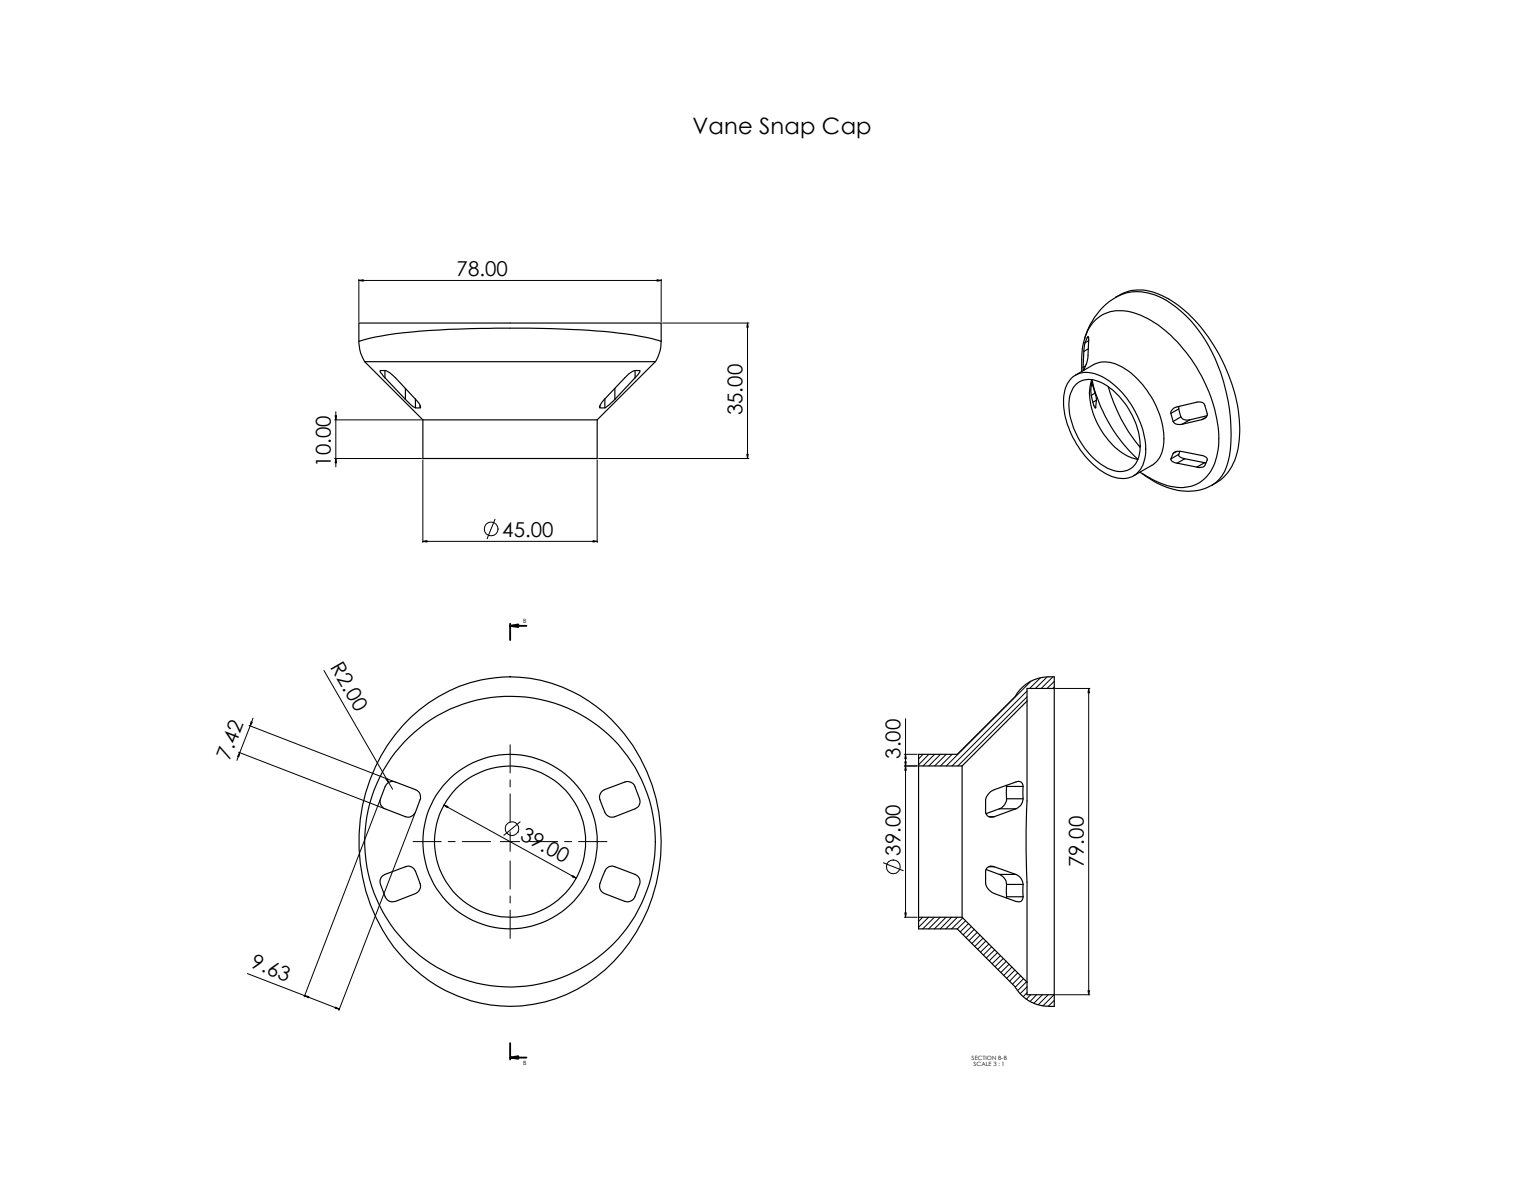
ISO-10303-21;
HEADER;
FILE_DESCRIPTION (('STEP AP214'),
    '1' );
FILE_NAME ('Vane Snap Cap.step',
    '2026-10-18T20:16:25',
    ( '' ),
    ( '' ),
    'SwSTEP 2.0',
    'SolidWorks 2025',
    '' );
FILE_SCHEMA (( 'AUTOMOTIVE_DESIGN' ));
ENDSEC;

DATA;
#5=CARTESIAN_POINT ( 'NONE',  ( -18.15804816958924306, -34.11099862341368549, 27.50000000000000000 ) ) ;
#9=CARTESIAN_POINT ( 'NONE',  ( -8.101746394734353984, -38.49011865887880646, 34.49999999999998579 ) ) ;
#19=CARTESIAN_POINT ( 'NONE',  ( 24.39344986792568903, -29.07448411189255211, 27.50000000000001066 ) ) ;
#42=EDGE_CURVE ( 'NONE', #19602, #22873, #7666, .T. ) ;
#47=CARTESIAN_POINT ( 'NONE',  ( 36.14613918203227172, 16.01870328439765601, 34.83083827288849221 ) ) ;
#98=CARTESIAN_POINT ( 'NONE',  ( -37.93368909164158254, 9.961195697873989729, 34.97277436636965575 ) ) ;
#131=CARTESIAN_POINT ( 'NONE',  ( 23.21352257770656635, -10.78826658734920052, 45.15942333309103418 ) ) ;
#132=ORIENTED_EDGE ( 'NONE', *, *, #23307, .F. ) ;
#138=AXIS2_PLACEMENT_3D ( 'NONE', #523, #22041, #27196 ) ;
#155=CARTESIAN_POINT ( 'NONE',  ( -7.108788511070779137, -38.72574257930638453, 34.49999999999999289 ) ) ;
#165=VERTEX_POINT ( 'NONE', #8736 ) ;
#166=CARTESIAN_POINT ( 'NONE',  ( 22.55938241427807256, 30.80590877286595841, 27.50000000000000355 ) ) ;
#170=DIRECTION ( 'NONE',  ( -0.000000000000000000, -0.000000000000000000, 1.000000000000000000 ) ) ;
#171=CARTESIAN_POINT ( 'NONE',  ( -30.03865005752669148, 15.52610542268208604, 41.18623755349101856 ) ) ;
#177=ORIENTED_EDGE ( 'NONE', *, *, #24246, .F. ) ;
#188=CARTESIAN_POINT ( 'NONE',  ( 27.51850911855329329, 30.14776422306135117, 30.03356538881464743 ) ) ;
#215=CARTESIAN_POINT ( 'NONE',  ( 24.35970437652574105, 13.37404834226503958, 47.21042702067963859 ) ) ;
#217=CARTESIAN_POINT ( 'NONE',  ( 19.49999999999992539, 1.626584906615178899E-14, 62.49999999999999289 ) ) ;
#224=B_SPLINE_CURVE_WITH_KNOTS ( 'NONE', 3,
 ( #24253, #10067, #7738, #5394 ),
 .UNSPECIFIED., .F., .F.,
 ( 4, 4 ),
 ( 2.143643656977390230E-07, 0.003421830178490235883 ),
 .UNSPECIFIED. ) ;
#247=CARTESIAN_POINT ( 'NONE',  ( -36.79585557548701757, 7.262324983800692912, 37.49999999996946087 ) ) ;
#254=VERTEX_POINT ( 'NONE', #21492 ) ;
#289=CARTESIAN_POINT ( 'NONE',  ( -32.19782014694307293, -14.25394737442115733, 39.78814634291943264 ) ) ;
#295=CARTESIAN_POINT ( 'NONE',  ( 25.24511578250132260, -28.23443549260979779, 34.49999999999999289 ) ) ;
#303=DIRECTION ( 'NONE',  ( 0.9329908884337535513, 0.3598999890241665334, 0.000000000000000000 ) ) ;
#309=CARTESIAN_POINT ( 'NONE',  ( -8.593763153356288598, -38.36129777999322954, 34.49999999999998579 ) ) ;
#338=CARTESIAN_POINT ( 'NONE',  ( 37.49999999999997158, 1.387778780781445676E-14, 37.50000000000000000 ) ) ;
#344=CARTESIAN_POINT ( 'NONE',  ( 30.96653510607171711, 25.84892707844779736, 34.59766498189470241 ) ) ;
#361=CARTESIAN_POINT ( 'NONE',  ( -23.13350093726293366, 11.03024450687078861, 49.37167574286524996 ) ) ;
#365=ORIENTED_EDGE ( 'NONE', *, *, #16572, .F. ) ;
#403=CARTESIAN_POINT ( 'NONE',  ( 29.61203839202722676, 15.40012917324034092, 41.62281023987512185 ) ) ;
#404=CARTESIAN_POINT ( 'NONE',  ( -34.20659985760524080, -15.57190080006868271, 37.50000000004849454 ) ) ;
#438=VERTEX_POINT ( 'NONE', #18642 ) ;
#441=CARTESIAN_POINT ( 'NONE',  ( -26.81381729043377504, 6.366069288663346093, 47.44085139292785414 ) ) ;
#451=CARTESIAN_POINT ( 'NONE',  ( 5.060094141397912360, 42.14075867279367316, 28.87075318537527835 ) ) ;
#457=CARTESIAN_POINT ( 'NONE',  ( -37.32236259411956780, 12.59516552021271885, 31.74041422182562755 ) ) ;
#490=CARTESIAN_POINT ( 'NONE',  ( 34.70577939417254498, 10.49309206032065944, 34.49999999999999289 ) ) ;
#492=CARTESIAN_POINT ( 'NONE',  ( 30.03792366816882975, 15.52577997660843145, 41.18702913624200335 ) ) ;
#501=CARTESIAN_POINT ( 'NONE',  ( -24.35970437652574105, -13.37404834226503070, 47.21042702067970254 ) ) ;
#505=CARTESIAN_POINT ( 'NONE',  ( 34.07302093592694803, 20.85404585400097233, 34.70738523996037372 ) ) ;
#506=FACE_OUTER_BOUND ( 'NONE', #20914, .T. ) ;
#519=CARTESIAN_POINT ( 'NONE',  ( -10.95918588188520282, 37.64010906258869227, 34.49999999999998579 ) ) ;
#523=CARTESIAN_POINT ( 'NONE',  ( 24.44496207165490276, 7.595930209050162141, -16.55003854064094426 ) ) ;
#526=VERTEX_POINT ( 'NONE', #217 ) ;
#548=CARTESIAN_POINT ( 'NONE',  ( -32.31395967786516366, -23.80510233529698993, 30.69444703814347264 ) ) ;
#551=EDGE_CURVE ( 'NONE', #10953, #254, #7134, .T. ) ;
#587=EDGE_CURVE ( 'NONE', #12561, #19716, #26583, .T. ) ;
#591=CARTESIAN_POINT ( 'NONE',  ( 35.02974205252522211, 18.72736911740413746, 31.20071108243496738 ) ) ;
#598=CARTESIAN_POINT ( 'NONE',  ( -19.51604255644980412, 36.82188910226315670, 29.35984054749004102 ) ) ;
#603=B_SPLINE_CURVE_WITH_KNOTS ( 'NONE', 3,
 ( #9449, #13968, #2105, #21117 ),
 .UNSPECIFIED., .F., .F.,
 ( 4, 4 ),
 ( 0.002976194933398900420, 0.003711256114093792156 ),
 .UNSPECIFIED. ) ;
#627=FACE_OUTER_BOUND ( 'NONE', #19855, .T. ) ;
#631=VECTOR ( 'NONE', #12349, 1000.000000000000000 ) ;
#639=CARTESIAN_POINT ( 'NONE',  ( -34.70577939417217550, -10.49309206032214270, 34.49999999999999289 ) ) ;
#641=CARTESIAN_POINT ( 'NONE',  ( 33.50775388423620882, 10.82565592554877121, 39.78708271175815270 ) ) ;
#643=CARTESIAN_POINT ( 'NONE',  ( 26.12638453225886792, 6.310846377660611850, 48.12226976367801257 ) ) ;
#646=ORIENTED_EDGE ( 'NONE', *, *, #6616, .F. ) ;
#654=CARTESIAN_POINT ( 'NONE',  ( -23.21352257770656990, 10.78826658734919519, 45.15942333309111234 ) ) ;
#665=ORIENTED_EDGE ( 'NONE', *, *, #13448, .F. ) ;
#672=DIRECTION ( 'NONE',  ( 0.000000000000000000, 0.000000000000000000, 1.000000000000000000 ) ) ;
#673=AXIS2_PLACEMENT_3D ( 'NONE', #16914, #18794, #7091 ) ;
#691=ADVANCED_FACE ( 'NONE', ( #10356 ), #20168, .F. ) ;
#704=CARTESIAN_POINT ( 'NONE',  ( -23.18616900178304974, -34.18096212676299217, 29.62072393548881877 ) ) ;
#711=B_SPLINE_SURFACE_WITH_KNOTS ( 'NONE', 3, 1, ( 
 ( #29500, #24966 ),
 ( #10153, #22316 ),
 ( #12970, #26861 ),
 ( #19658, #19825 ),
 ( #29347, #17492 ),
 ( #14986, #8137 ),
 ( #24498, #17804 ),
 ( #8288, #19982 ),
 ( #27013, #3144 ),
 ( #22160, #10468 ),
 ( #22462, #1109 ),
 ( #3602, #784 ),
 ( #13124, #18259 ),
 ( #11231, #13728 ),
 ( #25438, #4063 ),
 ( #25586, #13590 ),
 ( #6246, #3761 ),
 ( #8739, #20888 ),
 ( #1268, #1716 ),
 ( #28075, #25729 ),
 ( #13882, #4358 ),
 ( #11397, #10776 ),
 ( #4204, #20290 ),
 ( #29817, #23067 ),
 ( #8905, #23219 ),
 ( #1579, #27470 ),
 ( #11086, #8459 ),
 ( #17959, #22774 ),
 ( #15601, #25119 ),
 ( #18429, #1873 ),
 ( #8599, #18107 ),
 ( #30107, #3924 ),
 ( #27622, #15755 ),
 ( #25276, #20582 ) ),
 .UNSPECIFIED., .F., .F., .F.,
 ( 4, 2, 2, 2, 2, 2, 2, 2, 2, 2, 2, 2, 2, 2, 2, 2, 4 ),
 ( 2, 2 ),
 ( 0.000000000000000000, 0.06250000000000008327, 0.1250000000000001388, 0.1875000000000001943, 0.2500000000000002220, 0.3125000000000002220, 0.3750000000000002776, 0.4375000000000002776, 0.5000000000000003331, 0.5625000000000003331, 0.6250000000000002220, 0.6875000000000002220, 0.7500000000000002220, 0.8125000000000002220, 0.8750000000000001110, 0.9375000000000001110, 1.000000000000000000 ),
 ( 0.000000000000000000, 1.000000000000000000 ),
 .UNSPECIFIED. ) ;
#718=ORIENTED_EDGE ( 'NONE', *, *, #23326, .F. ) ;
#727=CARTESIAN_POINT ( 'NONE',  ( -1.248051566150084613, -39.49999999999997158, 27.49999999999999289 ) ) ;
#738=CARTESIAN_POINT ( 'NONE',  ( 0.000000000000000000, 39.50000000000000000, 27.50000000000000355 ) ) ;
#744=CARTESIAN_POINT ( 'NONE',  ( -27.80440265630350538, 29.80991922482741785, 30.06891749665959779 ) ) ;
#745=CARTESIAN_POINT ( 'NONE',  ( 77.99999999999998579, 42.50000000000000711, 27.50000000000000711 ) ) ;
#749=CARTESIAN_POINT ( 'NONE',  ( 27.81206575847386375, -25.09777039261014053, 34.50000000000000711 ) ) ;
#772=EDGE_LOOP ( 'NONE', ( #4852, #18862, #30452, #1067 ) ) ;
#776=CARTESIAN_POINT ( 'NONE',  ( 24.35970437652574105, 13.37404834226503958, -16.55003854064094426 ) ) ;
#784=CARTESIAN_POINT ( 'NONE',  ( -31.18890335284658732, 19.89223002944919116, 27.50000000000001066 ) ) ;
#786=CARTESIAN_POINT ( 'NONE',  ( 30.86161751192252822, 15.46691422980913266, 40.47962024281689963 ) ) ;
#790=CARTESIAN_POINT ( 'NONE',  ( 26.58938213246210580, 6.321715805855840031, 47.66948656093867243 ) ) ;
#807=EDGE_CURVE ( 'NONE', #6797, #17083, #20091, .T. ) ;
#824=CARTESIAN_POINT ( 'NONE',  ( -15.61095767114878541, 35.65786817450091206, 34.50000000000000000 ) ) ;
#838=EDGE_CURVE ( 'NONE', #18044, #17963, #995, .T. ) ;
#842=LINE ( 'NONE', #3035, #21019 ) ;
#846=VECTOR ( 'NONE', #2060, 1000.000000000000000 ) ;
#849=CARTESIAN_POINT ( 'NONE',  ( -23.21352257770656990, -10.78826658734919519, 45.15942333309109813 ) ) ;
#862=CARTESIAN_POINT ( 'NONE',  ( -34.80856967755993736, -19.21184172954434999, 31.15481810886020497 ) ) ;
#906=CARTESIAN_POINT ( 'NONE',  ( 27.03074382657074537, 6.449748410230989215, -16.55003854064094426 ) ) ;
#918=CARTESIAN_POINT ( 'NONE',  ( -38.56714466680799802, -6.442804806652034699, 32.09716166004417914 ) ) ;
#942=EDGE_CURVE ( 'NONE', #28122, #2953, #17667, .T. ) ;
#948=CARTESIAN_POINT ( 'NONE',  ( 31.89304216768362821, -14.79375299452194170, 35.60059606544044186 ) ) ;
#954=CARTESIAN_POINT ( 'NONE',  ( 24.44496207165490276, 7.595930209050162141, 49.40206402021032517 ) ) ;
#956=CARTESIAN_POINT ( 'NONE',  ( 16.53285166946374929, 35.10262665635723778, 34.50000000000000000 ) ) ;
#960=CARTESIAN_POINT ( 'NONE',  ( 30.74147208807243103, 15.49548351932574874, 40.57409041152969564 ) ) ;
#961=ORIENTED_EDGE ( 'NONE', *, *, #13499, .F. ) ;
#965=CARTESIAN_POINT ( 'NONE',  ( 33.50775388423620882, 10.82565592554877121, 35.54444202463886882 ) ) ;
#975=CARTESIAN_POINT ( 'NONE',  ( 77.99999999999998579, -42.50000000000001421, 27.50000000000000711 ) ) ;
#976=CARTESIAN_POINT ( 'NONE',  ( 7.864568376310370645, 41.74085412114251881, 28.90542812248210325 ) ) ;
#979=CARTESIAN_POINT ( 'NONE',  ( 26.12638453225886792, 6.310846377660614515, 43.87962907655873579 ) ) ;
#989=CARTESIAN_POINT ( 'NONE',  ( -33.70208146031188789, 13.89198562565741923, 34.49999999999999289 ) ) ;
#995=B_SPLINE_CURVE_WITH_KNOTS ( 'NONE', 3,
 ( #11129, #20628, #30146, #15962, #30750, #9393, #21536, #24028, #23883, #14206, #14058, #171, #16252, #4861 ),
 .UNSPECIFIED., .F., .F.,
 ( 4, 2, 2, 2, 2, 2, 4 ),
 ( 2.111077618484504239E-07, 0.0004668847438969890226, 0.0009335583800321295943, 0.001400232016167270166, 0.001866905652302410738, 0.002800252924572703590, 0.003733600196842996443 ),
 .UNSPECIFIED. ) ;
#1006=EDGE_CURVE ( 'NONE', #20257, #22873, #4629, .T. ) ;
#1025=EDGE_CURVE ( 'NONE', #30101, #30448, #12431, .T. ) ;
#1026=CARTESIAN_POINT ( 'NONE',  ( -28.50858587296695745, -29.13344744256045615, 30.13847653714394070 ) ) ;
#1031=DIRECTION ( 'NONE',  ( -0.9329908884337535513, 0.3598999890241665334, 0.000000000000000000 ) ) ;
#1039=CIRCLE ( 'NONE', #2525, 19.49999999999996447 ) ;
#1048=VERTEX_POINT ( 'NONE', #5486 ) ;
#1067=ORIENTED_EDGE ( 'NONE', *, *, #3732, .F. ) ;
#1071=CARTESIAN_POINT ( 'NONE',  ( 25.56256718580103637, -32.12586005794658206, 29.82918954436054193 ) ) ;
#1103=CARTESIAN_POINT ( 'NONE',  ( -33.01877980957529957, 12.12572312222180493, 39.84356070656661331 ) ) ;
#1109=CARTESIAN_POINT ( 'NONE',  ( -28.55068628633582861, 24.19494186940698199, 27.50000000000001066 ) ) ;
#1117=LINE ( 'NONE', #9899, #29855 ) ;
#1125=CARTESIAN_POINT ( 'NONE',  ( 13.29126524260693998, 35.08562276291469573, 37.49999999993516298 ) ) ;
#1127=CARTESIAN_POINT ( 'NONE',  ( 24.44496207165490276, 7.595930209050162141, 45.15942333309104129 ) ) ;
#1129=DIRECTION ( 'NONE',  ( 1.000000000000000000, 0.000000000000000000, 0.000000000000000000 ) ) ;
#1144=FACE_OUTER_BOUND ( 'NONE', #21557, .T. ) ;
#1169=CARTESIAN_POINT ( 'NONE',  ( 24.35970437652574105, 13.37404834226503958, 42.96778633356035471 ) ) ;
#1179=CARTESIAN_POINT ( 'NONE',  ( -15.55309275218070830, -34.20504001467671884, 37.49999999988268229 ) ) ;
#1201=CARTESIAN_POINT ( 'NONE',  ( 33.26787633654601706, -9.290711110048576415, 40.45924760685198862 ) ) ;
#1203=VERTEX_POINT ( 'NONE', #29467 ) ;
#1210=EDGE_CURVE ( 'NONE', #27501, #29565, #30630, .T. ) ;
#1218=CARTESIAN_POINT ( 'NONE',  ( -4.163336342344337027E-14, 1.387778780781445676E-14, 37.50000000000000000 ) ) ;
#1229=CARTESIAN_POINT ( 'NONE',  ( -24.35970437652574105, 13.37404834226503247, 42.96778633356043287 ) ) ;
#1233=DIRECTION ( 'NONE',  ( 1.000000000000000000, 0.000000000000000000, 0.000000000000000000 ) ) ;
#1268=CARTESIAN_POINT ( 'NONE',  ( -35.76481447503398670, -5.202797454133643917, 34.80090346875804386 ) ) ;
#1269=CARTESIAN_POINT ( 'NONE',  ( 30.33183837007556249, 13.53414739637283226, -16.55003854064094426 ) ) ;
#1280=B_SPLINE_CURVE_WITH_KNOTS ( 'NONE', 3,
 ( #2307, #12145, #11993, #11834, #4507, #21164, #4800, #28524, #26026, #24132, #7155, #9957, #441, #2624 ),
 .UNSPECIFIED., .F., .F.,
 ( 4, 2, 2, 2, 2, 2, 4 ),
 ( 2.108610145898612731E-07, 0.0004867403503157787643, 0.0009732698396169676622, 0.001459799328918156506, 0.001946328818219345350, 0.002919387796821717399, 0.003892446775424089015 ),
 .UNSPECIFIED. ) ;
#1285=CARTESIAN_POINT ( 'NONE',  ( 19.84998497291395125, 36.59036391654254317, 29.38252776222237372 ) ) ;
#1287=CARTESIAN_POINT ( 'NONE',  ( -33.51229671200703564, -9.872960191568498800, 35.82118098709739940 ) ) ;
#1288=CARTESIAN_POINT ( 'NONE',  ( -33.48612972047447300, 10.91418318924902131, 39.78046893947538365 ) ) ;
#1296=CARTESIAN_POINT ( 'NONE',  ( 9.743151247090292344, -38.04912300944125292, 27.50000000000000000 ) ) ;
#1307=CARTESIAN_POINT ( 'NONE',  ( -24.44496207165490276, -7.595930209050158588, 49.40206402021039622 ) ) ;
#1309=B_SPLINE_CURVE_WITH_KNOTS ( 'NONE', 3,
 ( #28103, #25755, #20466, #11254 ),
 .UNSPECIFIED., .F., .F.,
 ( 4, 4 ),
 ( 3.022186913359086288E-07, 0.007932103869840195776 ),
 .UNSPECIFIED. ) ;
#1321=CARTESIAN_POINT ( 'NONE',  ( 27.86235613436985759, 14.72519157938689460, 39.24389099736750808 ) ) ;
#1326=CARTESIAN_POINT ( 'NONE',  ( -11.70595374688322821, -40.54787758647957219, 34.56692815348143455 ) ) ;
#1334=CARTESIAN_POINT ( 'NONE',  ( 31.89304216768362821, -14.79375299452194348, 39.84323675255973995 ) ) ;
#1336=ORIENTED_EDGE ( 'NONE', *, *, #9963, .T. ) ;
#1343=B_SPLINE_CURVE_WITH_KNOTS ( 'NONE', 3,
 ( #28708, #11874, #19499, #9676, #12175, #21673, #26843, #5148, #14659, #4840, #24161, #2813, #12336, #26205, #17153, #7650, #26672, #19039, #19641, #2509, #29011, #23697, #14510, #28553, #4998, #309, #9, #155, #7799, #14355, #12023, #7185, #23865, #21836 ),
 .UNSPECIFIED., .F., .F.,
 ( 4, 2, 2, 2, 2, 2, 2, 2, 2, 2, 2, 2, 2, 2, 2, 2, 4 ),
 ( 0.1877422973930296390, 0.1907727015327729259, 0.1938031056725162127, 0.1998639139520027586, 0.2028943180917460454, 0.2044095201616177027, 0.2059247222314893322, 0.2119855305109759058, 0.2150159346507191649, 0.2165311367205908222, 0.2180463387904624517, 0.2241071470699490531, 0.2271375512096923677, 0.2286527532795639972, 0.2301679553494356545, 0.2331983594891789413, 0.2362287636289222559 ),
 .UNSPECIFIED. ) ;
#1371=CARTESIAN_POINT ( 'NONE',  ( -5.974369479646943759, 42.02548368003539991, 34.60052964640640738 ) ) ;
#1384=CARTESIAN_POINT ( 'NONE',  ( 12.58101777923778997, -40.23389158998374171, 29.03989791324179848 ) ) ;
#1398=CARTESIAN_POINT ( 'NONE',  ( 35.99999999999999289, -2.601438916704202242, 34.80090346875810070 ) ) ;
#1412=CARTESIAN_POINT ( 'NONE',  ( 24.44496207165490276, -7.595930209050162141, -16.55003854064094426 ) ) ;
#1414=CARTESIAN_POINT ( 'NONE',  ( -33.43088607478084384, -9.613432587296607323, 40.21452297281935984 ) ) ;
#1439=ORIENTED_EDGE ( 'NONE', *, *, #14389, .F. ) ;
#1448=CYLINDRICAL_SURFACE ( 'NONE', #28363, 19.49999999999996447 ) ;
#1450=ORIENTED_EDGE ( 'NONE', *, *, #13936, .F. ) ;
#1452=CARTESIAN_POINT ( 'NONE',  ( -33.42925964089141644, -11.06161099612212695, 35.54550565580013455 ) ) ;
#1455=CARTESIAN_POINT ( 'NONE',  ( -33.42925964089140933, 11.06161099612212695, 39.78814634291943264 ) ) ;
#1474=PLANE ( 'NONE',  #26220 ) ;
#1483=CARTESIAN_POINT ( 'NONE',  ( 35.71656808851346199, -17.11898487263705704, 31.35097916509175420 ) ) ;
#1497=CARTESIAN_POINT ( 'NONE',  ( -31.10273980501929003, -15.38400267427140022, 40.30072466179765911 ) ) ;
#1511=CARTESIAN_POINT ( 'NONE',  ( 33.51208342369033488, -9.877893692955346694, 40.06259746622173168 ) ) ;
#1518=ORIENTED_EDGE ( 'NONE', *, *, #17633, .T. ) ;
#1526=CARTESIAN_POINT ( 'NONE',  ( -29.61203839202723032, -15.40012917324033381, 37.38016955275590192 ) ) ;
#1535=EDGE_LOOP ( 'NONE', ( #14556, #8831 ) ) ;
#1545=CARTESIAN_POINT ( 'NONE',  ( 17.94248964168179583, 34.33858135081683827, 34.80090346875809360 ) ) ;
#1547=ORIENTED_EDGE ( 'NONE', *, *, #7279, .F. ) ;
#1553=ORIENTED_EDGE ( 'NONE', *, *, #27298, .F. ) ;
#1558=CARTESIAN_POINT ( 'NONE',  ( 23.13152334643393715, 11.98019263786950184, 48.95036236640387983 ) ) ;
#1563=B_SPLINE_CURVE_WITH_KNOTS ( 'NONE', 3,
 ( #8926, #25745, #9067, #30722, #30123, #1889 ),
 .UNSPECIFIED., .F., .F.,
 ( 4, 2, 4 ),
 ( 0.01057608626842624147, 0.01589305904737019909, 0.02121003182631415324 ),
 .UNSPECIFIED. ) ;
#1575=CARTESIAN_POINT ( 'NONE',  ( 33.48319591361583036, 9.771272583783428445, 40.12028472023447279 ) ) ;
#1579=CARTESIAN_POINT ( 'NONE',  ( -23.69412710310941605, -29.84645176427128987, 34.80090346875804386 ) ) ;
#1597=EDGE_CURVE ( 'NONE', #6797, #18116, #28187, .T. ) ;
#1604=CARTESIAN_POINT ( 'NONE',  ( -33.03011559203990544, 8.976883822286589876, 40.77182279851235336 ) ) ;
#1607=ORIENTED_EDGE ( 'NONE', *, *, #15669, .T. ) ;
#1631=ORIENTED_EDGE ( 'NONE', *, *, #838, .F. ) ;
#1634=CARTESIAN_POINT ( 'NONE',  ( 35.57581530336350539, -17.46952725568587894, 34.79368316662617389 ) ) ;
#1636=VECTOR ( 'NONE', #26633, 1000.000000000000000 ) ;
#1669=CIRCLE ( 'NONE', #19099, 37.50000000000001421 ) ;
#1680=CARTESIAN_POINT ( 'NONE',  ( 31.34809375791739683, -25.29209928965034848, 30.54052050932160256 ) ) ;
#1681=DIRECTION ( 'NONE',  ( -0.000000000000000000, -0.000000000000000000, -1.000000000000000000 ) ) ;
#1698=CARTESIAN_POINT ( 'NONE',  ( -30.33183837007556249, -13.53414739637282516, -16.55003854064094426 ) ) ;
#1702=LINE ( 'NONE', #20570, #17967 ) ;
#1704=CARTESIAN_POINT ( 'NONE',  ( -23.07950435457407679, 11.50806656539752737, -16.55003854064094426 ) ) ;
#1708=ORIENTED_EDGE ( 'NONE', *, *, #23072, .F. ) ;
#1716=CARTESIAN_POINT ( 'NONE',  ( -35.76481447503398670, -5.202797454133643917, 27.50000000000000355 ) ) ;
#1733=ADVANCED_FACE ( 'NONE', ( #5565 ), #29631, .F. ) ;
#1734=CARTESIAN_POINT ( 'NONE',  ( 26.11179934312167816, -14.04991663536889135, 41.10667063058289727 ) ) ;
#1764=CARTESIAN_POINT ( 'NONE',  ( 32.19782014694307293, 14.25394737442116444, -16.55003854064094426 ) ) ;
#1775=CARTESIAN_POINT ( 'NONE',  ( 36.88240865182195449, -7.258209409195951700, 37.49999999993649880 ) ) ;
#1778=ORIENTED_EDGE ( 'NONE', *, *, #6616, .T. ) ;
#1784=VERTEX_POINT ( 'NONE', #4948 ) ;
#1786=CARTESIAN_POINT ( 'NONE',  ( -6.388525611213331068, -41.95271539343359990, 34.59875978651353989 ) ) ;
#1795=CARTESIAN_POINT ( 'NONE',  ( 23.07601128794333434, 11.40611796340042261, 45.01673140500131609 ) ) ;
#1802=CARTESIAN_POINT ( 'NONE',  ( 24.35970437652574816, -13.37404834226503958, 47.21042702067961727 ) ) ;
#1810=ORIENTED_EDGE ( 'NONE', *, *, #27747, .F. ) ;
#1823=ORIENTED_EDGE ( 'NONE', *, *, #26337, .F. ) ;
#1828=CARTESIAN_POINT ( 'NONE',  ( 29.61203839202725518, -15.40012917324033381, 41.62281023987508632 ) ) ;
#1839=CIRCLE ( 'NONE', #27764, 37.50000000000001421 ) ;
#1848=CARTESIAN_POINT ( 'NONE',  ( 17.94248964168179583, -34.33858135081684537, 34.80090346875808649 ) ) ;
#1873=CARTESIAN_POINT ( 'NONE',  ( -11.52197458429825261, -37.50933785548060229, 27.49999999999999645 ) ) ;
#1888=CARTESIAN_POINT ( 'NONE',  ( 0.000000000000000000, 42.50000000000000000, 37.50000000000000000 ) ) ;
#1889=CARTESIAN_POINT ( 'NONE',  ( 34.70577939417254498, 10.49309206032065944, 34.49999999999999289 ) ) ;
#1890=CARTESIAN_POINT ( 'NONE',  ( 24.35970437652574816, -13.37404834226503958, 47.21042702067961727 ) ) ;
#1920=DIRECTION ( 'NONE',  ( -0.3598999890241700306, 0.9329908884337522190, 0.000000000000000000 ) ) ;
#1926=CARTESIAN_POINT ( 'NONE',  ( 27.05998495714042207, -30.73416682267111000, 34.52243346884028341 ) ) ;
#1948=ORIENTED_EDGE ( 'NONE', *, *, #3915, .T. ) ;
#1949=CARTESIAN_POINT ( 'NONE',  ( 33.56327786402390245, -10.34181101807379477, 35.63689980405263924 ) ) ;
#1963=EDGE_LOOP ( 'NONE', ( #27185, #1518, #15732, #5340 ) ) ;
#1980=CARTESIAN_POINT ( 'NONE',  ( 2.212236613306092892, 42.53911549472210396, 34.61403848092495394 ) ) ;
#1982=FACE_OUTER_BOUND ( 'NONE', #21567, .T. ) ;
#1984=CARTESIAN_POINT ( 'NONE',  ( -26.58597676761596063, 6.321098805557481271, 43.43030304422423882 ) ) ;
#1986=EDGE_LOOP ( 'NONE', ( #7812, #6825, #5779, #9715, #22803 ) ) ;
#1988=CARTESIAN_POINT ( 'NONE',  ( 25.53015708495998837, -6.470147010658197750, 44.42018155122899969 ) ) ;
#1992=DIRECTION ( 'NONE',  ( -0.7071067811865487940, -8.659560562354948882E-17, -0.7071067811865463515 ) ) ;
#2006=ORIENTED_EDGE ( 'NONE', *, *, #838, .T. ) ;
#2007=CARTESIAN_POINT ( 'NONE',  ( 24.44496207165490631, -7.595930209050163029, 45.15942333309103418 ) ) ;
#2022=ORIENTED_EDGE ( 'NONE', *, *, #29111, .F. ) ;
#2024=CARTESIAN_POINT ( 'NONE',  ( 2.049713242724727991, -39.50000000000001421, 34.50000000000000000 ) ) ;
#2049=CARTESIAN_POINT ( 'NONE',  ( 29.73573388937572659, -22.26985569269989895, 27.49999999999999645 ) ) ;
#2060=DIRECTION ( 'NONE',  ( -0.000000000000000000, -0.000000000000000000, 1.000000000000000000 ) ) ;
#2070=CARTESIAN_POINT ( 'NONE',  ( 8.813079928575357158, -41.51132794799057280, 28.92494092171985898 ) ) ;
#2082=CARTESIAN_POINT ( 'NONE',  ( -31.79204601741444236, -14.90874471747207686, 39.88609648712696298 ) ) ;
#2094=B_SPLINE_CURVE_WITH_KNOTS ( 'NONE', 3,
 ( #6785, #6951, #25974, #23611, #11774, #21275, #18965, #28473, #3192, #19882, #5682, #10516, #29236, #15178 ),
 .UNSPECIFIED., .F., .F.,
 ( 4, 2, 2, 2, 2, 2, 4 ),
 ( 2.980251112064282051E-07, 0.0007442722521831233746, 0.001488246479255040311, 0.001860233592791005501, 0.002232220706326970474, 0.002604207819862935230, 0.002976194933398900420 ),
 .UNSPECIFIED. ) ;
#2102=CARTESIAN_POINT ( 'NONE',  ( -23.72845085825479572, 12.99428747377816151, 43.70389027930196590 ) ) ;
#2103=EDGE_CURVE ( 'NONE', #7486, #17105, #15760, .T. ) ;
#2105=CARTESIAN_POINT ( 'NONE',  ( 33.51937758206383222, -10.82799271170304323, 35.53333982454045525 ) ) ;
#2120=PLANE ( 'NONE',  #11256 ) ;
#2122=CARTESIAN_POINT ( 'NONE',  ( -33.54031841762500932, 21.84949147252275381, 30.89863097042385931 ) ) ;
#2146=CARTESIAN_POINT ( 'NONE',  ( 11.52197458429827037, 37.50933785548059518, 34.80090346875809360 ) ) ;
#2157=EDGE_LOOP ( 'NONE', ( #5767, #21097, #13023 ) ) ;
#2159=DIRECTION ( 'NONE',  ( 0.000000000000000000, 0.000000000000000000, 1.000000000000000000 ) ) ;
#2163=EDGE_CURVE ( 'NONE', #20389, #2236, #1117, .T. ) ;
#2172=PLANE ( 'NONE',  #6139 ) ;
#2175=CARTESIAN_POINT ( 'NONE',  ( -23.07950435457404481, 11.62838985844542883, 49.15679243825150024 ) ) ;
#2187=B_SPLINE_CURVE_WITH_KNOTS ( 'NONE', 3,
 ( #14332, #21037, #12156, #21655, #9052, #7167, #18872, #23529, #14485, #14171, #2175, #21497 ),
 .UNSPECIFIED., .F., .F.,
 ( 4, 2, 2, 2, 2, 4 ),
 ( 2.975096543306551241E-07, 0.0007805422437037903925, 0.001560786977753250097, 0.002341031711802709584, 0.002731154078827434124, 0.003121276445852158229 ),
 .UNSPECIFIED. ) ;
#2203=CARTESIAN_POINT ( 'NONE',  ( 32.30280224124133781, 17.44315250269476891, 27.50000000000000711 ) ) ;
#2225=CARTESIAN_POINT ( 'NONE',  ( 24.72409811164068572, 32.98527725324579052, 29.74032444299796296 ) ) ;
#2236=VERTEX_POINT ( 'NONE', #22859 ) ;
#2251=CARTESIAN_POINT ( 'NONE',  ( -23.13391957319673864, -11.02874123662317984, 49.37194155098371340 ) ) ;
#2271=CARTESIAN_POINT ( 'NONE',  ( -23.13757476351621989, 34.33072287895263486, 34.50373710099040636 ) ) ;
#2307=CARTESIAN_POINT ( 'NONE',  ( -24.44496207165490276, 7.595930209050158588, 49.40206402021040333 ) ) ;
#2308=ORIENTED_EDGE ( 'NONE', *, *, #9530, .F. ) ;
#2310=EDGE_CURVE ( 'NONE', #20027, #22947, #13896, .T. ) ;
#2312=EDGE_CURVE ( 'NONE', #18831, #12912, #21331, .T. ) ;
#2321=CARTESIAN_POINT ( 'NONE',  ( -9.534095299299449877, -41.21642526093817338, 28.95179448440414660 ) ) ;
#2326=CARTESIAN_POINT ( 'NONE',  ( 19.07166558422281355, -33.51611795593300513, 34.49999999999998579 ) ) ;
#2329=CARTESIAN_POINT ( 'NONE',  ( -33.42925964089140933, 11.06161099612212695, 35.54550565580014876 ) ) ;
#2333=FACE_OUTER_BOUND ( 'NONE', #1535, .T. ) ;
#2337=CARTESIAN_POINT ( 'NONE',  ( -34.94982008328430823, 9.785536899246608300, 27.50000000000000355 ) ) ;
#2341=ORIENTED_EDGE ( 'NONE', *, *, #15669, .F. ) ;
#2346=EDGE_CURVE ( 'NONE', #2236, #27891, #22862, .T. ) ;
#2347=DIRECTION ( 'NONE',  ( -0.000000000000000000, -0.000000000000000000, 1.000000000000000000 ) ) ;
#2353=UNCERTAINTY_MEASURE_WITH_UNIT (LENGTH_MEASURE( 1.000000000000000082E-05 ), #10820, 'distance_accuracy_value', 'NONE');
#2358=CARTESIAN_POINT ( 'NONE',  ( 9.775490391764725118, 38.10998157767718908, 27.50000000000000355 ) ) ;
#2387=CARTESIAN_POINT ( 'NONE',  ( 31.22614026363978112, 25.47088236078499079, 30.52195406502089980 ) ) ;
#2398=CARTESIAN_POINT ( 'NONE',  ( -30.38302862529102910, -15.53680216053817986, 36.63232123326689305 ) ) ;
#2410=CARTESIAN_POINT ( 'NONE',  ( -23.21352257770656990, -10.78826658734919519, 45.15942333309109813 ) ) ;
#2421=DIRECTION ( 'NONE',  ( 0.000000000000000000, 0.000000000000000000, 1.000000000000000000 ) ) ;
#2443=CARTESIAN_POINT ( 'NONE',  ( -31.96854311794286474, 24.49685236950227463, 34.62152949131530022 ) ) ;
#2445=CARTESIAN_POINT ( 'NONE',  ( 23.62400240902268322, 9.724154461249522541, 45.23564988763768469 ) ) ;
#2446=B_SPLINE_CURVE_WITH_KNOTS ( 'NONE', 3,
 ( #5245, #24262, #12427, #21922 ),
 .UNSPECIFIED., .F., .F.,
 ( 4, 4 ),
 ( 2.143643656977390230E-07, 0.003421830178490235016 ),
 .UNSPECIFIED. ) ;
#2462=CARTESIAN_POINT ( 'NONE',  ( 9.268856789657291984, 38.25380398711768493, 27.50000000000001066 ) ) ;
#2463=ORIENTED_EDGE ( 'NONE', *, *, #23072, .T. ) ;
#2468=EDGE_LOOP ( 'NONE', ( #9610, #11994, #13861, #1439 ) ) ;
#2470=B_SPLINE_CURVE_WITH_KNOTS ( 'NONE', 3,
 ( #8363, #17879, #22679, #1334, #15830, #22993, #11007, #30030, #23304, #30472, #9114, #20658, #25810, #23447 ),
 .UNSPECIFIED., .F., .F.,
 ( 4, 2, 2, 2, 2, 2, 4 ),
 ( 2.111077618454142872E-07, 0.0004668847438969826258, 0.0009335583800321198365, 0.001400232016167257156, 0.001866905652302394258, 0.002800252924572680605, 0.003733600196842966519 ),
 .UNSPECIFIED. ) ;
#2486=CARTESIAN_POINT ( 'NONE',  ( -11.99928012101186958, -40.44431291024729092, 29.02086326041609254 ) ) ;
#2492=CARTESIAN_POINT ( 'NONE',  ( 23.62400240902267967, -9.724154461249520764, 45.23564988763767758 ) ) ;
#2499=CARTESIAN_POINT ( 'NONE',  ( -4.163336342344337027E-14, 1.387778780781445676E-14, 52.50000000000000000 ) ) ;
#2504=CARTESIAN_POINT ( 'NONE',  ( -34.41394710506926202, -11.60896409125851036, 27.50000000000000355 ) ) ;
#2509=CARTESIAN_POINT ( 'NONE',  ( -18.27078283711139051, -34.03626749931920159, 34.50000000000000000 ) ) ;
#2521=CARTESIAN_POINT ( 'NONE',  ( 31.51879050643202618, 19.12242388295294404, 27.49999999999999645 ) ) ;
#2525=AXIS2_PLACEMENT_3D ( 'NONE', #23977, #2159, #9494 ) ;
#2544=CARTESIAN_POINT ( 'NONE',  ( 37.44001822671184243, 11.96995332997097705, 31.77506326509126922 ) ) ;
#2564=CARTESIAN_POINT ( 'NONE',  ( -24.44496207165490276, -7.595930209050158588, 45.15942333309111234 ) ) ;
#2566=ORIENTED_EDGE ( 'NONE', *, *, #21422, .T. ) ;
#2586=CARTESIAN_POINT ( 'NONE',  ( -27.03074382657074537, 6.449748410230984774, -16.55003854064094426 ) ) ;
#2595=CARTESIAN_POINT ( 'NONE',  ( -37.69406220750976644, 10.98234033417770128, 31.84368292284955260 ) ) ;
#2611=CARTESIAN_POINT ( 'NONE',  ( -29.61203839202723032, 15.40012917324033204, 41.62281023987520001 ) ) ;
#2624=CARTESIAN_POINT ( 'NONE',  ( -27.03074382657074537, 6.449748410230984774, 47.21042702067971675 ) ) ;
#2630=CARTESIAN_POINT ( 'NONE',  ( 32.06000616748023901, 24.34448380653289234, 30.63959652465332439 ) ) ;
#2634=CARTESIAN_POINT ( 'NONE',  ( -20.51889442710595191, -36.16778909624833460, 29.42346760871654965 ) ) ;
#2638=ORIENTED_EDGE ( 'NONE', *, *, #21576, .T. ) ;
#2643=CARTESIAN_POINT ( 'NONE',  ( 31.56327786402390245, 10.34181101807379655, -16.55003854064094426 ) ) ;
#2667=CARTESIAN_POINT ( 'NONE',  ( -24.44496207165490276, 7.595930209050158588, -16.55003854064094426 ) ) ;
#2692=CARTESIAN_POINT ( 'NONE',  ( 37.14755456718950910, 5.754233978929971904, 37.49999999992148503 ) ) ;
#2709=CARTESIAN_POINT ( 'NONE',  ( -24.50428919468314959, -7.442132857256927636, 45.14840622132437886 ) ) ;
#2733=CARTESIAN_POINT ( 'NONE',  ( -32.60829997825918980, -13.18983524832147936, 35.60092001944732232 ) ) ;
#2743=FACE_BOUND ( 'NONE', #20323, .T. ) ;
#2751=CARTESIAN_POINT ( 'NONE',  ( -26.39612953643615256, 31.29397724899363809, 29.91504862403774467 ) ) ;
#2753=CARTESIAN_POINT ( 'NONE',  ( -29.61203839202723032, -15.40012917324033381, 41.62281023987518580 ) ) ;
#2793=PLANE ( 'NONE',  #12044 ) ;
#2812=ORIENTED_EDGE ( 'NONE', *, *, #4404, .T. ) ;
#2813=CARTESIAN_POINT ( 'NONE',  ( -27.19745787981435825, -25.87981526613175021, 34.49999999999998579 ) ) ;
#2833=CARTESIAN_POINT ( 'NONE',  ( 25.41654339919795902, 6.509636863629522097, 48.76343458312116041 ) ) ;
#2847=CARTESIAN_POINT ( 'NONE',  ( 38.96845262021057010, 1.827616164893528961, 32.22212046549758924 ) ) ;
#2857=VERTEX_POINT ( 'NONE', #6209 ) ;
#2864=CARTESIAN_POINT ( 'NONE',  ( -8.026378865559991027, 38.50914575096116010, 34.49999999999998579 ) ) ;
#2874=ORIENTED_EDGE ( 'NONE', *, *, #26738, .F. ) ;
#2884=B_SPLINE_CURVE_WITH_KNOTS ( 'NONE', 3,
 ( #25506, #3824, #27686, #13349, #16136, #4129, #25653, #4270, #13798, #23299, #2709, #19085 ),
 .UNSPECIFIED., .F., .F.,
 ( 4, 2, 2, 2, 2, 4 ),
 ( 2.975219550372212526E-07, 0.0009689891316535818779, 0.001937680741352126390, 0.002906372351050671120, 0.003390718155899948363, 0.003875063960749225173 ),
 .UNSPECIFIED. ) ;
#2890=CARTESIAN_POINT ( 'NONE',  ( 29.61203839202723032, 15.40012917324034092, 37.38016955275583797 ) ) ;
#2898=FACE_BOUND ( 'NONE', #13547, .T. ) ;
#2909=CARTESIAN_POINT ( 'NONE',  ( -39.06789089969338846, -0.5117148525053366592, 32.25338167081577012 ) ) ;
#2910=ORIENTED_EDGE ( 'NONE', *, *, #3708, .T. ) ;
#2911=CARTESIAN_POINT ( 'NONE',  ( -33.42925964089140933, 11.06161099612212695, -16.55003854064094426 ) ) ;
#2938=EDGE_CURVE ( 'NONE', #15816, #23899, #5708, .T. ) ;
#2953=VERTEX_POINT ( 'NONE', #20547 ) ;
#2955=CARTESIAN_POINT ( 'NONE',  ( 10.11194158890137729, 41.13960854804319212, 28.95784450080078898 ) ) ;
#2961=CARTESIAN_POINT ( 'NONE',  ( -29.46596134976465109, 27.84982784967258240, 30.27354135555054171 ) ) ;
#2972=CARTESIAN_POINT ( 'NONE',  ( 27.03074382657074537, -6.449748410230991880, 47.21042702067962438 ) ) ;
#2982=VERTEX_POINT ( 'NONE', #7132 ) ;
#2991=CARTESIAN_POINT ( 'NONE',  ( 29.03395105464274195, 23.44066905138924284, 34.50000000000000000 ) ) ;
#3013=CARTESIAN_POINT ( 'NONE',  ( -23.07950435457408034, -11.74770253185616298, 44.86091080599459247 ) ) ;
#3018=ORIENTED_EDGE ( 'NONE', *, *, #23926, .F. ) ;
#3030=LINE ( 'NONE', #27197, #25696 ) ;
#3035=CARTESIAN_POINT ( 'NONE',  ( -4.776122516674677878E-15, -42.50000000000000000, 37.50000000000000000 ) ) ;
#3046=ORIENTED_EDGE ( 'NONE', *, *, #14327, .F. ) ;
#3047=PRODUCT_CONTEXT ( 'NONE', #24920, 'mechanical' ) ;
#3054=CARTESIAN_POINT ( 'NONE',  ( -24.74483793516321484, -32.88075240386160658, 29.75196967776350832 ) ) ;
#3058=B_SPLINE_CURVE_WITH_KNOTS ( 'NONE', 3,
 ( #5346, #19221, #7387, #21710 ),
 .UNSPECIFIED., .F., .F.,
 ( 4, 4 ),
 ( 3.018024802580205417E-07, 0.007932103453629112816 ),
 .UNSPECIFIED. ) ;
#3084=CARTESIAN_POINT ( 'NONE',  ( -24.42252949794886163, -29.12958095736449593, 27.50000000000000355 ) ) ;
#3098=CARTESIAN_POINT ( 'NONE',  ( 25.20647278166642735, 28.20479727972634265, 27.50000000000001066 ) ) ;
#3101=CARTESIAN_POINT ( 'NONE',  ( 38.98831344968873935, -1.224499394254795703, 32.22844543117250993 ) ) ;
#3107=CARTESIAN_POINT ( 'NONE',  ( -36.55886824564901616, 15.02606788761555379, 31.54031350539812806 ) ) ;
#3109=CARTESIAN_POINT ( 'NONE',  ( -24.35970437652574105, -13.37404834226503070, 42.96778633356041865 ) ) ;
#3113=CARTESIAN_POINT ( 'NONE',  ( 32.02497887436175006, -18.15461798050466413, 34.49999999999999289 ) ) ;
#3126=DIRECTION ( 'NONE',  ( -0.3598999890241658117, -0.9329908884337538844, 0.000000000000000000 ) ) ;
#3135=CARTESIAN_POINT ( 'NONE',  ( -33.42925964089140933, 11.06161099612212695, 39.78814634291943264 ) ) ;
#3136=CARTESIAN_POINT ( 'NONE',  ( -24.85846090629200589, 6.933313039714898984, 44.95040115368838229 ) ) ;
#3144=CARTESIAN_POINT ( 'NONE',  ( -23.69412710310941961, 29.84645176427129698, 27.50000000000001066 ) ) ;
#3147=CARTESIAN_POINT ( 'NONE',  ( -25.88640477275121299, -6.345529225273951468, 48.34755156421752531 ) ) ;
#3163=ORIENTED_EDGE ( 'NONE', *, *, #21544, .F. ) ;
#3168=VERTEX_POINT ( 'NONE', #3533 ) ;
#3185=VERTEX_POINT ( 'NONE', #23452 ) ;
#3192=CARTESIAN_POINT ( 'NONE',  ( 33.41032657756569080, -9.567127522732027600, 36.00434311239766316 ) ) ;
#3206=CARTESIAN_POINT ( 'NONE',  ( -34.24553848958673541, -20.37971379545431105, 31.04075131429937073 ) ) ;
#3223=CARTESIAN_POINT ( 'NONE',  ( 19.49999999999992539, 1.626584906615178899E-14, 62.49999999999999289 ) ) ;
#3230=CARTESIAN_POINT ( 'NONE',  ( -35.98785884342813546, 1.199078351611056137, 27.50000000000001066 ) ) ;
#3240=LINE ( 'NONE', #906, #8862 ) ;
#3241=VERTEX_POINT ( 'NONE', #15992 ) ;
#3247=CARTESIAN_POINT ( 'NONE',  ( -29.06340618096728434, 28.34784734514725812, 30.22145900126884754 ) ) ;
#3248=CARTESIAN_POINT ( 'NONE',  ( -4.776122516674677878E-15, -42.50000000000000000, 32.26246401786215046 ) ) ;
#3267=EDGE_CURVE ( 'NONE', #8258, #29295, #30236, .T. ) ;
#3274=CARTESIAN_POINT ( 'NONE',  ( 27.03074382657074537, 6.449748410230989215, 47.21042702067963148 ) ) ;
#3286=CARTESIAN_POINT ( 'NONE',  ( 5.090001874368171642, 39.11868163644495411, 34.49999999999999289 ) ) ;
#3288=CARTESIAN_POINT ( 'NONE',  ( -35.89043209166185022, -3.548455793344783338, 34.73498294778838869 ) ) ;
#3290=CARTESIAN_POINT ( 'NONE',  ( 31.10273980501927227, 15.38400267427140200, 40.30072466179758806 ) ) ;
#3292=CARTESIAN_POINT ( 'NONE',  ( -24.44496207165490276, -7.595930209050158588, 49.40206402021039622 ) ) ;
#3307=CARTESIAN_POINT ( 'NONE',  ( 5.060094141397912360, 42.14075867279367316, 28.87075318537528190 ) ) ;
#3310=EDGE_CURVE ( 'NONE', #526, #16582, #9751, .T. ) ;
#3312=CARTESIAN_POINT ( 'NONE',  ( -33.48610676296128474, -10.91424270342314529, 35.53783135159724793 ) ) ;
#3316=EDGE_CURVE ( 'NONE', #7486, #18819, #13809, .T. ) ;
#3322=CARTESIAN_POINT ( 'NONE',  ( -9.996178806698672759, 37.96205643617683023, 34.49999999999998579 ) ) ;
#3323=B_SPLINE_CURVE_WITH_KNOTS ( 'NONE', 3,
 ( #17499, #22325, #965, #29507, #8144, #20735 ),
 .UNSPECIFIED., .F., .F.,
 ( 4, 2, 4 ),
 ( 2.111164903073641161E-07, 0.0003706953849294931068, 0.0007411796533686788348 ),
 .UNSPECIFIED. ) ;
#3331=CARTESIAN_POINT ( 'NONE',  ( -25.07950435457407323, -11.50806656539752737, -16.55003854064094426 ) ) ;
#3347=CARTESIAN_POINT ( 'NONE',  ( -0.2228332965694262147, -42.50627663705900261, 28.83920636888621658 ) ) ;
#3357=CARTESIAN_POINT ( 'NONE',  ( -32.76876142772501055, -23.05949818548782915, 34.65609885376971278 ) ) ;
#3363=DIRECTION ( 'NONE',  ( 0.3598999890241665334, 0.9329908884337535513, 0.000000000000000000 ) ) ;
#3366=ORIENTED_EDGE ( 'NONE', *, *, #22090, .F. ) ;
#3381=CARTESIAN_POINT ( 'NONE',  ( 35.86437274510301165, -3.536632535698085000, 34.72985588596458939 ) ) ;
#3389=VECTOR ( 'NONE', #28499, 1000.000000000000000 ) ;
#3390=CARTESIAN_POINT ( 'NONE',  ( -35.57943149391982018, 6.143871028500258902, 27.50000000000000711 ) ) ;
#3432=MANIFOLD_SOLID_BREP ( 'Fillet1', #26783 ) ;
#3444=EDGE_CURVE ( 'NONE', #23323, #8258, #3030, .T. ) ;
#3455=CARTESIAN_POINT ( 'NONE',  ( 31.79204601741444947, 14.90874471747209107, 39.88609648712689904 ) ) ;
#3466=CARTESIAN_POINT ( 'NONE',  ( -24.02316098943739675, -13.21662147465773707, 47.58119960047616814 ) ) ;
#3473=CARTESIAN_POINT ( 'NONE',  ( 10.34195653711237739, 41.08375821880306233, 34.57657180301586664 ) ) ;
#3479=FACE_OUTER_BOUND ( 'NONE', #22300, .T. ) ;
#3499=VERTEX_POINT ( 'NONE', #19777 ) ;
#3503=CARTESIAN_POINT ( 'NONE',  ( 3.648422002868280778, 32.24090100849873863, 28.87075318537527480 ) ) ;
#3508=CARTESIAN_POINT ( 'NONE',  ( -32.28307784207223108, 8.475829241206282560, 37.38016955275591613 ) ) ;
#3521=ORIENTED_EDGE ( 'NONE', *, *, #9530, .T. ) ;
#3525=CARTESIAN_POINT ( 'NONE',  ( -18.69039966852829693, -32.51582865032699488, 37.49999999996209255 ) ) ;
#3532=CARTESIAN_POINT ( 'NONE',  ( 30.50204315964899493, 15.53056155674292071, 36.52918211141452787 ) ) ;
#3533=CARTESIAN_POINT ( 'NONE',  ( -4.375757216953428294E-15, -39.50000000000000000, 27.50000000000000355 ) ) ;
#3534=LINE ( 'NONE', #13198, #25242 ) ;
#3540=CARTESIAN_POINT ( 'NONE',  ( 32.44949699048085989, -8.540025205420066712, 41.44554437670149127 ) ) ;
#3563=CARTESIAN_POINT ( 'NONE',  ( 8.890978711956464053, -41.40418588057009686, 28.93512758870527790 ) ) ;
#3602=CARTESIAN_POINT ( 'NONE',  ( -31.18890335284658732, 19.89223002944919116, 34.80090346875805096 ) ) ;
#3620=CARTESIAN_POINT ( 'NONE',  ( 18.96813378833590846, 37.14367329901003245, 34.51897858957566001 ) ) ;
#3621=PRODUCT_DEFINITION ( 'UNKNOWN', '', #23831, #30100 ) ;
#3625=CARTESIAN_POINT ( 'NONE',  ( 32.19782014694307293, 14.25394737442116444, 39.78814634291936159 ) ) ;
#3626=CARTESIAN_POINT ( 'NONE',  ( 25.07950435457407323, -11.50806656539753270, -16.55003854064094426 ) ) ;
#3632=EDGE_CURVE ( 'NONE', #17044, #7581, #5794, .T. ) ;
#3634=B_SPLINE_CURVE_WITH_KNOTS ( 'NONE', 3,
 ( #20918, #9082, #18600, #6732, #1296, #3791, #10810, #20324, #28414, #25763, #9387, #19196, #18905, #19, #4544, #11571, #23878, #18743, #11887, #2049, #14051, #4394, #30588, #7039, #14944, #4853, #14201, #23557, #12034, #24454, #21211, #11720, #21527, #21382, #30741, #13913, #9227, #16706, #9685, #28721, #28259, #19048, #2203, #2521, #16547, #26066, #16400, #4697, #3098, #23709, #14369, #166, #25915, #7774, #6885, #21065, #12616, #9532, #5441, #17283, #2358, #22109, #28565, #7194, #26216, #26815, #19769, #738 ),
 .UNSPECIFIED., .F., .F.,
 ( 4, 2, 2, 2, 2, 2, 2, 2, 2, 2, 2, 2, 2, 2, 2, 2, 2, 2, 2, 2, 2, 2, 2, 2, 2, 2, 2, 2, 2, 2, 2, 2, 2, 4 ),
 ( 0.000000000000000000, 0.007385865967851777160, 0.01107879895177766617, 0.01477173193570355432, 0.02215759790355534276, 0.02400406439551829724, 0.02585053088748124478, 0.02954346387140714680, 0.03323639685533304883, 0.03508286334729599637, 0.03692932983925895085, 0.04431519580711074102, 0.04616166229907370244, 0.04800812879103664998, 0.05170106177496255201, 0.05908692774281434912, 0.06093339423477729666, 0.06277986072674023033, 0.06647279371066613929, 0.07385865967851792946, 0.07570512617048090476, 0.07755159266244385230, 0.08124452564636976126, 0.08863039161422160694, 0.09047685810618456836, 0.09232332459814752978, 0.09601625758207343875, 0.09970919056599936159, 0.1015556570579623091, 0.1034021235499252567, 0.1107879895177770330, 0.1144809225017029281, 0.1163273889936658617, 0.1181738554856288231 ),
 .UNSPECIFIED. ) ;
#3655=CARTESIAN_POINT ( 'NONE',  ( -33.18396177295070260, 9.163667207889121258, 36.33144972432103970 ) ) ;
#3673=DIRECTION ( 'NONE',  ( 0.000000000000000000, 0.000000000000000000, 1.000000000000000000 ) ) ;
#3681=DIRECTION ( 'NONE',  ( -0.3598999890241650346, 0.9329908884337541064, 0.000000000000000000 ) ) ;
#3694=CARTESIAN_POINT ( 'NONE',  ( 33.55224573311711822, -10.10291939066353351, 39.95985515795820930 ) ) ;
#3708=EDGE_CURVE ( 'NONE', #17083, #8115, #14138, .T. ) ;
#3711=VERTEX_POINT ( 'NONE', #13852 ) ;
#3715=CARTESIAN_POINT ( 'NONE',  ( -10.80934979336458746, 35.92737112411883516, 37.49999999999869971 ) ) ;
#3732=EDGE_CURVE ( 'NONE', #12560, #30628, #22769, .T. ) ;
#3735=CARTESIAN_POINT ( 'NONE',  ( 21.86019681245146629, -31.48592878035298170, 34.80090346875810781 ) ) ;
#3745=CARTESIAN_POINT ( 'NONE',  ( 24.14277784031759566, 13.29036922066994642, 47.44085139300341325 ) ) ;
#3748=CARTESIAN_POINT ( 'NONE',  ( -33.56830061431172396, -10.30497729095454851, 39.88583012291989149 ) ) ;
#3761=CARTESIAN_POINT ( 'NONE',  ( -36.00000000000000000, 2.601438916704200466, 27.50000000000000355 ) ) ;
#3765=CARTESIAN_POINT ( 'NONE',  ( 32.28307784207223108, 8.475829241206289666, 37.38016955275583086 ) ) ;
#3773=CARTESIAN_POINT ( 'NONE',  ( 31.56327786402390245, 10.34181101807379655, -16.55003854064094426 ) ) ;
#3791=CARTESIAN_POINT ( 'NONE',  ( 12.09913007902929216, -37.22566656357093962, 27.50000000000001421 ) ) ;
#3796=VECTOR ( 'NONE', #18793, 1000.000000000000000 ) ;
#3812=CARTESIAN_POINT ( 'NONE',  ( -0.2184780646694884920, -42.50603693459091659, 34.61341353021254008 ) ) ;
#3821=DIRECTION ( 'NONE',  ( 1.000000000000000000, 0.000000000000000000, -0.000000000000000000 ) ) ;
#3822=CARTESIAN_POINT ( 'NONE',  ( -21.00812534432329315, -35.81422794740934279, 29.45837907140124656 ) ) ;
#3824=CARTESIAN_POINT ( 'NONE',  ( -26.81368379037234817, -6.366017791192965625, 43.19835251265433840 ) ) ;
#3858=EDGE_LOOP ( 'NONE', ( #22277, #29955, #23055, #7847, #12844, #22784, #6492, #17892, #1547 ) ) ;
#3865=CARTESIAN_POINT ( 'NONE',  ( -16.30640546663167356, 38.61508539432780651, 34.53478415730283757 ) ) ;
#3867=CARTESIAN_POINT ( 'NONE',  ( 24.35970437652574816, -13.37404834226503958, 47.21042702067961727 ) ) ;
#3873=ORIENTED_EDGE ( 'NONE', *, *, #2310, .F. ) ;
#3875=ADVANCED_FACE ( 'NONE', ( #5254 ), #26152, .F. ) ;
#3878=CARTESIAN_POINT ( 'NONE',  ( 14.37255012589468883, -39.51473361311175125, 29.10561451833818225 ) ) ;
#3890=CARTESIAN_POINT ( 'NONE',  ( 15.85884089648730289, -35.55173462727349687, 27.50000000000000355 ) ) ;
#3915=EDGE_CURVE ( 'NONE', #26574, #5509, #26442, .T. ) ;
#3924=CARTESIAN_POINT ( 'NONE',  ( -4.677126025380971441, -39.24912351428226742, 27.49999999999999645 ) ) ;
#3943=CARTESIAN_POINT ( 'NONE',  ( 24.14264434021281858, -13.29031772318284865, 47.44099319989518193 ) ) ;
#3949=ORIENTED_EDGE ( 'NONE', *, *, #942, .F. ) ;
#3960=CARTESIAN_POINT ( 'NONE',  ( -32.60829997825918980, 13.18983524832148291, 35.60092001944733653 ) ) ;
#3974=CARTESIAN_POINT ( 'NONE',  ( 27.38650679510956820, -30.38832073129480094, 30.00757695512932344 ) ) ;
#4012=CARTESIAN_POINT ( 'NONE',  ( -30.03792366816883330, -15.52577997660842435, 36.94438844912276920 ) ) ;
#4014=CARTESIAN_POINT ( 'NONE',  ( -3.917446247819842409, 37.31292274963767142, 37.50000000001976019 ) ) ;
#4033=CARTESIAN_POINT ( 'NONE',  ( 34.83396020575241891, 10.30249279383515848, 34.80090346875810070 ) ) ;
#4049=CARTESIAN_POINT ( 'NONE',  ( -32.68377466358848693, -8.668986135640256663, 41.18623755341147330 ) ) ;
#4063=CARTESIAN_POINT ( 'NONE',  ( -34.83396020575242602, 10.30249279383516381, 27.50000000000001066 ) ) ;
#4082=FACE_OUTER_BOUND ( 'NONE', #16701, .T. ) ;
#4100=CARTESIAN_POINT ( 'NONE',  ( 33.01877980957530667, -12.12572312222180670, 39.84356070656651383 ) ) ;
#4107=VERTEX_POINT ( 'NONE', #8063 ) ;
#4118=CARTESIAN_POINT ( 'NONE',  ( 36.29469092165690114, -9.775717669454033754, 37.49999999999255351 ) ) ;
#4123=ORIENTED_EDGE ( 'NONE', *, *, #2310, .T. ) ;
#4127=CARTESIAN_POINT ( 'NONE',  ( -15.78417422266179315, -38.97739145708682429, 29.15446067280243270 ) ) ;
#4129=CARTESIAN_POINT ( 'NONE',  ( -25.41654339919794836, -6.509636863629521208, 44.52079389600195469 ) ) ;
#4144=CARTESIAN_POINT ( 'NONE',  ( 0.8476314135585345522, 42.50000000000000711, 28.83974596215562869 ) ) ;
#4164=VERTEX_POINT ( 'NONE', #1802 ) ;
#4165=DIRECTION ( 'NONE',  ( -0.9329908884337522190, -0.3598999890241700306, 0.000000000000000000 ) ) ;
#4179=CARTESIAN_POINT ( 'NONE',  ( -4.776122516674677878E-15, -42.50000000000000000, 28.83974596215560737 ) ) ;
#4180=CARTESIAN_POINT ( 'NONE',  ( 4.677126025380961671, -39.24912351428227453, 27.50000000000000355 ) ) ;
#4181=VERTEX_POINT ( 'NONE', #28319 ) ;
#4189=DIRECTION ( 'NONE',  ( 1.000000000000000000, 0.000000000000000000, 0.000000000000000000 ) ) ;
#4194=ADVANCED_FACE ( 'NONE', ( #6944 ), #8983, .F. ) ;
#4204=CARTESIAN_POINT ( 'NONE',  ( -31.18890335284659443, -19.89223002944918051, 34.80090346875804386 ) ) ;
#4222=CARTESIAN_POINT ( 'NONE',  ( -27.99175947355483274, 24.84200504376626029, 27.50000000000000355 ) ) ;
#4253=EDGE_CURVE ( 'NONE', #16582, #17083, #21587, .T. ) ;
#4255=CARTESIAN_POINT ( 'NONE',  ( -33.52485258639264032, 10.76172163581451890, 35.54788606881927393 ) ) ;
#4259=CARTESIAN_POINT ( 'NONE',  ( 14.08068486978915601, -39.64040334357339646, 29.09405787692634249 ) ) ;
#4265=FACE_OUTER_BOUND ( 'NONE', #16896, .T. ) ;
#4270=CARTESIAN_POINT ( 'NONE',  ( -24.86084284002701850, -6.930828199065642181, 44.94877300773892159 ) ) ;
#4277=CARTESIAN_POINT ( 'NONE',  ( 23.13152334643393715, 11.98019263786950184, 44.70772167928459595 ) ) ;
#4280=DIRECTION ( 'NONE',  ( 0.000000000000000000, 0.000000000000000000, 1.000000000000000000 ) ) ;
#4308=CARTESIAN_POINT ( 'NONE',  ( -10.19388640336980068, 41.04980642620002840, 28.96642789899617298 ) ) ;
#4324=CARTESIAN_POINT ( 'NONE',  ( -35.37867965644041135, 9.545149127882528772E-15, 35.37867965644034740 ) ) ;
#4333=CARTESIAN_POINT ( 'NONE',  ( 2.338573377552013888, -39.50000000000001421, 34.80090346875810070 ) ) ;
#4339=AXIS2_PLACEMENT_3D ( 'NONE', #16684, #26506, #21185 ) ;
#4340=CYLINDRICAL_SURFACE ( 'NONE', #24606, 2.000000000000001776 ) ;
#4341=CARTESIAN_POINT ( 'NONE',  ( 23.15418787629628739, 10.94208358504856804, 49.39104550112972447 ) ) ;
#4349=DIRECTION ( 'NONE',  ( -0.000000000000000000, -0.000000000000000000, 1.000000000000000000 ) ) ;
#4358=CARTESIAN_POINT ( 'NONE',  ( -34.13832859401785669, -12.80067323710187921, 27.49999999999998934 ) ) ;
#4362=B_SPLINE_CURVE_WITH_KNOTS ( 'NONE', 3,
 ( #22847, #15985, #6164, #8667, #25805, #11308, #13947, #1497, #20945, #15827, #4437, #2082, #6475, #8809, #23141, #30027 ),
 .UNSPECIFIED., .F., .F.,
 ( 4, 2, 2, 2, 2, 2, 2, 4 ),
 ( 2.980374332640320740E-07, 0.0009280375596593464730, 0.001391907320772394928, 0.001855777081885443165, 0.002319646842998491186, 0.002783516604111547447, 0.003247386365224603274, 0.003711256126337659968 ),
 .UNSPECIFIED. ) ;
#4363=DIRECTION ( 'NONE',  ( 0.3598999890241668664, -0.9329908884337534403, 0.000000000000000000 ) ) ;
#4365=CARTESIAN_POINT ( 'NONE',  ( -4.375757216953428294E-15, -39.50000000000000000, 34.49999999999999289 ) ) ;
#4375=DIRECTION ( 'NONE',  ( 0.000000000000000000, 0.000000000000000000, 1.000000000000000000 ) ) ;
#4386=ORIENTED_EDGE ( 'NONE', *, *, #11639, .F. ) ;
#4394=CARTESIAN_POINT ( 'NONE',  ( 31.61035137122363636, -19.06714716585487679, 27.50000000000000355 ) ) ;
#4401=CARTESIAN_POINT ( 'NONE',  ( -32.19782014694307293, 14.25394737442115733, -16.55003854064094426 ) ) ;
#4402=CARTESIAN_POINT ( 'NONE',  ( 33.56327786402394509, -10.57885966092500674, 39.80973752444699443 ) ) ;
#4404=EDGE_CURVE ( 'NONE', #12912, #19716, #19764, .T. ) ;
#4410=ORIENTED_EDGE ( 'NONE', *, *, #12035, .F. ) ;
#4412=EDGE_CURVE ( 'NONE', #10675, #30448, #6746, .T. ) ;
#4415=FACE_OUTER_BOUND ( 'NONE', #28711, .T. ) ;
#4420=CARTESIAN_POINT ( 'NONE',  ( 14.71494672776318957, -39.36570965915668552, 29.11934627781901952 ) ) ;
#4425=CARTESIAN_POINT ( 'NONE',  ( 24.35970437652574105, 13.37404834226503958, -16.55003854064094426 ) ) ;
#4437=CARTESIAN_POINT ( 'NONE',  ( -31.57476163834523675, -15.10795358447669301, 39.99718304312881401 ) ) ;
#4462=DIRECTION ( 'NONE',  ( -0.000000000000000000, -0.000000000000000000, 1.000000000000000000 ) ) ;
#4478=CARTESIAN_POINT ( 'NONE',  ( -37.02637947441376554, 5.976920169802977689, 37.50000000003053913 ) ) ;
#4485=CARTESIAN_POINT ( 'NONE',  ( 24.85846090629200589, -6.933313039714902537, 44.95040115368828992 ) ) ;
#4500=ADVANCED_FACE ( 'NONE', ( #13487 ), #1474, .F. ) ;
#4507=CARTESIAN_POINT ( 'NONE',  ( -24.85846090629201299, 6.933313039714896320, 49.19304184080765907 ) ) ;
#4527=PLANE ( 'NONE',  #12134 ) ;
#4529=CARTESIAN_POINT ( 'NONE',  ( -23.08950671686661948, 11.27322061222802851, 45.06306679229680157 ) ) ;
#4531=CARTESIAN_POINT ( 'NONE',  ( -26.45199234830066004, 26.79642899342907825, 27.50000000000000355 ) ) ;
#4544=CARTESIAN_POINT ( 'NONE',  ( 25.24607261983683060, -28.18396486040856530, 27.50000000000000355 ) ) ;
#4562=CARTESIAN_POINT ( 'NONE',  ( -25.07950435457407323, 11.50806656539752737, -16.55003854064094426 ) ) ;
#4570=CARTESIAN_POINT ( 'NONE',  ( 13.83399314246956813, -39.74420824290464793, 34.55195916885559626 ) ) ;
#4593=EDGE_LOOP ( 'NONE', ( #24402, #19731, #27523, #18874 ) ) ;
#4600=ADVANCED_FACE ( 'NONE', ( #24185 ), #23889, .F. ) ;
#4602=DIRECTION ( 'NONE',  ( 1.000000000000000000, 0.000000000000000000, 0.000000000000000000 ) ) ;
#4622=CARTESIAN_POINT ( 'NONE',  ( -36.61847497238780846, 14.68214248103183905, 31.56314805174072191 ) ) ;
#4624=LINE ( 'NONE', #2911, #18830 ) ;
#4627=CARTESIAN_POINT ( 'NONE',  ( 32.44940373544195467, 8.539989232413363496, 37.20300302271262183 ) ) ;
#4629=B_SPLINE_CURVE_WITH_KNOTS ( 'NONE', 3,
 ( #7522, #10012, #641, #10470, #24180, #10310 ),
 .UNSPECIFIED., .F., .F.,
 ( 4, 2, 4 ),
 ( 2.111164903090458206E-07, 0.0003706953849294946247, 0.0007411796533686801358 ),
 .UNSPECIFIED. ) ;
#4633=CARTESIAN_POINT ( 'NONE',  ( 25.88604317058895532, -6.345278376181632041, 44.10533075955772375 ) ) ;
#4636=CARTESIAN_POINT ( 'NONE',  ( 27.03074382657074537, -6.449748410230991880, 47.21042702067962438 ) ) ;
#4637=CARTESIAN_POINT ( 'NONE',  ( -32.28307784207223108, -8.475829241206275455, -16.55003854064094426 ) ) ;
#4660=ORIENTED_EDGE ( 'NONE', *, *, #27298, .T. ) ;
#4675=DIRECTION ( 'NONE',  ( 1.000000000000000000, 0.000000000000000000, 0.000000000000000000 ) ) ;
#4683=CARTESIAN_POINT ( 'NONE',  ( -23.07950435457394889, 11.39182330144667432, 45.01971494674684493 ) ) ;
#4697=CARTESIAN_POINT ( 'NONE',  ( 25.62842000332392800, 27.74319361490436009, 27.50000000000001421 ) ) ;
#4702=B_SPLINE_CURVE_WITH_KNOTS ( 'NONE', 3,
 ( #6446, #16107, #3960, #6594 ),
 .UNSPECIFIED., .F., .F.,
 ( 4, 4 ),
 ( 2.143643656964903641E-07, 0.003421830178490235450 ),
 .UNSPECIFIED. ) ;
#4712=CARTESIAN_POINT ( 'NONE',  ( -23.62400240902268322, -9.724154461249517212, 49.47829057475703252 ) ) ;
#4720=CARTESIAN_POINT ( 'NONE',  ( 24.51012911669599958, 28.40691445806841386, 37.50000000005638157 ) ) ;
#4721=CARTESIAN_POINT ( 'NONE',  ( -4.163336342344337027E-14, 1.387778780781445676E-14, 62.49999999999999289 ) ) ;
#4722=ORIENTED_EDGE ( 'NONE', *, *, #21635, .T. ) ;
#4724=PLANE ( 'NONE',  #22159 ) ;
#4730=ORIENTED_EDGE ( 'NONE', *, *, #1597, .T. ) ;
#4749=CARTESIAN_POINT ( 'NONE',  ( 2.538591345309722414, 42.43983719188426562, 28.84490890740515567 ) ) ;
#4756=LINE ( 'NONE', #2586, #16068 ) ;
#4764=CARTESIAN_POINT ( 'NONE',  ( -27.01611617209707816, 30.66277435038324128, 34.52684288084092401 ) ) ;
#4766=DIRECTION ( 'NONE',  ( -0.000000000000000000, -0.000000000000000000, 1.000000000000000000 ) ) ;
#4770=AXIS2_PLACEMENT_3D ( 'NONE', #11070, #11217, #25258 ) ;
#4771=DIRECTION ( 'NONE',  ( 0.000000000000000000, 0.000000000000000000, 1.000000000000000000 ) ) ;
#4800=CARTESIAN_POINT ( 'NONE',  ( -25.18466322232232457, 6.657711795334223304, 48.95036236631857207 ) ) ;
#4806=EDGE_CURVE ( 'NONE', #17339, #20389, #18315, .T. ) ;
#4808=EDGE_CURVE ( 'NONE', #14021, #12560, #15981, .T. ) ;
#4812=EDGE_CURVE ( 'NONE', #19313, #19602, #3323, .T. ) ;
#4824=DIRECTION ( 'NONE',  ( -0.000000000000000000, -0.000000000000000000, 1.000000000000000000 ) ) ;
#4833=CARTESIAN_POINT ( 'NONE',  ( -16.56775953753748354, -35.09133156286775090, 27.50000000000001066 ) ) ;
#4840=CARTESIAN_POINT ( 'NONE',  ( -28.12430571491142572, -24.65851106883863508, 34.49999999999999289 ) ) ;
#4852=ORIENTED_EDGE ( 'NONE', *, *, #6683, .F. ) ;
#4853=CARTESIAN_POINT ( 'NONE',  ( 34.25977182215996919, -12.14538519402363903, 27.50000000000000000 ) ) ;
#4856=DIRECTION ( 'NONE',  ( -0.000000000000000000, -0.000000000000000000, 1.000000000000000000 ) ) ;
#4861=CARTESIAN_POINT ( 'NONE',  ( -29.61203839202723032, 15.40012917324033204, 41.62281023987520001 ) ) ;
#4878=CARTESIAN_POINT ( 'NONE',  ( 30.58308285076613586, 26.38567509859110061, 34.58766046687880902 ) ) ;
#4903=CARTESIAN_POINT ( 'NONE',  ( 32.28307784207223108, 8.475829241206289666, 37.38016955275583086 ) ) ;
#4904=ORIENTED_EDGE ( 'NONE', *, *, #8427, .F. ) ;
#4910=CARTESIAN_POINT ( 'NONE',  ( -23.59263552078001425, 12.85968412197262545, 43.88772444904758885 ) ) ;
#4911=CARTESIAN_POINT ( 'NONE',  ( -4.163336342344337027E-14, 1.387778780781445676E-14, 37.50000000000000000 ) ) ;
#4914=VERTEX_POINT ( 'NONE', #2329 ) ;
#4927=FACE_OUTER_BOUND ( 'NONE', #18242, .T. ) ;
#4931=CARTESIAN_POINT ( 'NONE',  ( -32.22095362587521095, 24.09752088550972005, 30.66525214441444902 ) ) ;
#4935=CARTESIAN_POINT ( 'NONE',  ( 33.51212652704789008, 9.877957833750135919, 35.81989857765422869 ) ) ;
#4948=CARTESIAN_POINT ( 'NONE',  ( 24.35970437652574105, 13.37404834226503958, 47.21042702067963859 ) ) ;
#4952=CARTESIAN_POINT ( 'NONE',  ( 4.677126025380971441, 39.24912351428226742, 34.80090346875809360 ) ) ;
#4971=ADVANCED_FACE ( 'NONE', ( #19334 ), #24151, .F. ) ;
#4995=CARTESIAN_POINT ( 'NONE',  ( -9.834155381565185650, -38.09377060189168418, 27.50000000000000355 ) ) ;
#4997=ADVANCED_FACE ( 'NONE', ( #7172 ), #14339, .F. ) ;
#4998=CARTESIAN_POINT ( 'NONE',  ( -10.05674029770914579, -37.94258163987278465, 34.49999999999998579 ) ) ;
#5035=CARTESIAN_POINT ( 'NONE',  ( 22.67433715982020459, 34.69950560126978445, 29.56729215824071488 ) ) ;
#5039=B_SPLINE_CURVE_WITH_KNOTS ( 'NONE', 3,
 ( #18982, #7588, #2445, #17089 ),
 .UNSPECIFIED., .F., .F.,
 ( 4, 4 ),
 ( 2.143643656977390230E-07, 0.003421830178490239353 ),
 .UNSPECIFIED. ) ;
#5060=ORIENTED_EDGE ( 'NONE', *, *, #4812, .F. ) ;
#5068=CARTESIAN_POINT ( 'NONE',  ( -23.16720440049831709, -10.90834004837188154, 49.39346268393973816 ) ) ;
#5082=VERTEX_POINT ( 'NONE', #7596 ) ;
#5087=CARTESIAN_POINT ( 'NONE',  ( -22.90437772071893363, 29.69852781866232760, 37.50000000002601297 ) ) ;
#5089=CARTESIAN_POINT ( 'NONE',  ( -24.35970437652574105, -13.37404834226503070, 47.21042702067970254 ) ) ;
#5103=CARTESIAN_POINT ( 'NONE',  ( -77.99999999999998579, -42.49999999999998579, 32.33822642395377045 ) ) ;
#5110=DIRECTION ( 'NONE',  ( 1.000000000000000000, 0.000000000000000000, 0.000000000000000000 ) ) ;
#5116=EDGE_LOOP ( 'NONE', ( #21681, #28520, #6220, #13437 ) ) ;
#5123=CARTESIAN_POINT ( 'NONE',  ( 23.07593096178833747, -11.40900259639455605, 45.01551998640317009 ) ) ;
#5124=ORIENTED_EDGE ( 'NONE', *, *, #7088, .F. ) ;
#5136=CARTESIAN_POINT ( 'NONE',  ( 34.17252016804844317, -12.46427775875993937, 34.49999999999999289 ) ) ;
#5148=CARTESIAN_POINT ( 'NONE',  ( -29.56528975567554696, -22.55618809495488009, 34.49999999999999289 ) ) ;
#5154=ORIENTED_EDGE ( 'NONE', *, *, #551, .F. ) ;
#5180=DIRECTION ( 'NONE',  ( -0.000000000000000000, -0.000000000000000000, 1.000000000000000000 ) ) ;
#5188=CARTESIAN_POINT ( 'NONE',  ( 38.93535427911099589, 2.534171857450247423, 35.07262524311201446 ) ) ;
#5196=VERTEX_POINT ( 'NONE', #29727 ) ;
#5237=ORIENTED_EDGE ( 'NONE', *, *, #16413, .T. ) ;
#5243=CARTESIAN_POINT ( 'NONE',  ( -37.84083111920662645, -10.30891341277128248, 34.96466318893187264 ) ) ;
#5245=CARTESIAN_POINT ( 'NONE',  ( -23.21352257770656990, 10.78826658734919519, 49.40206402021039622 ) ) ;
#5246=CARTESIAN_POINT ( 'NONE',  ( 33.36692087966583387, 9.471517865689168758, 36.07226619909889820 ) ) ;
#5254=FACE_OUTER_BOUND ( 'NONE', #14795, .T. ) ;
#5264=FACE_OUTER_BOUND ( 'NONE', #12664, .T. ) ;
#5281=DIRECTION ( 'NONE',  ( -0.1430297813019457409, -0.9897183850271336070, 0.000000000000000000 ) ) ;
#5285=DIRECTION ( 'NONE',  ( 0.9329908884337542174, -0.3598999890241648125, 0.000000000000000000 ) ) ;
#5299=DIRECTION ( 'NONE',  ( -0.000000000000000000, -0.000000000000000000, 1.000000000000000000 ) ) ;
#5311=CONICAL_SURFACE ( 'NONE', #30229, 35.37867965644036872, 0.7853981633974500554 ) ;
#5319=CARTESIAN_POINT ( 'NONE',  ( 12.86231920026284925, 36.90765539456646849, 34.50000000000000000 ) ) ;
#5338=CARTESIAN_POINT ( 'NONE',  ( 28.40292615218646688, 29.15708363699292249, 30.13690029699395012 ) ) ;
#5339=CARTESIAN_POINT ( 'NONE',  ( -36.00000000000000000, -1.100768691257133318E-12, 34.75735931288076586 ) ) ;
#5340=ORIENTED_EDGE ( 'NONE', *, *, #4808, .F. ) ;
#5346=CARTESIAN_POINT ( 'NONE',  ( 27.03074382657074182, -6.449748410230990991, 42.96778633356034049 ) ) ;
#5358=CARTESIAN_POINT ( 'NONE',  ( -33.53437127389221928, 14.37219272518421853, 34.49999999999999289 ) ) ;
#5362=EDGE_CURVE ( 'NONE', #16582, #526, #11846, .T. ) ;
#5367=DIRECTION ( 'NONE',  ( -0.000000000000000000, -0.000000000000000000, 1.000000000000000000 ) ) ;
#5369=AXIS2_PLACEMENT_3D ( 'NONE', #25176, #3673, #3821 ) ;
#5375=DIRECTION ( 'NONE',  ( 1.000000000000000000, 0.000000000000000000, 0.000000000000000000 ) ) ;
#5394=CARTESIAN_POINT ( 'NONE',  ( -23.21352257770656990, -10.78826658734919519, 45.15942333309109813 ) ) ;
#5399=CARTESIAN_POINT ( 'NONE',  ( -36.21276101124586688, -16.00154621764524165, 34.83087659172860384 ) ) ;
#5415=CARTESIAN_POINT ( 'NONE',  ( -4.776122516674677878E-15, -42.50000000000000000, 32.33822642395377045 ) ) ;
#5441=CARTESIAN_POINT ( 'NONE',  ( 14.91216081148350270, 35.95613889121786855, 27.50000000000000711 ) ) ;
#5449=CARTESIAN_POINT ( 'NONE',  ( -38.16194395454053989, 8.856611044372645125, 31.97620825923344512 ) ) ;
#5473=ORIENTED_EDGE ( 'NONE', *, *, #4253, .T. ) ;
#5475=CARTESIAN_POINT ( 'NONE',  ( 30.74201181684197337, -15.50830195949553314, 36.32560960729286847 ) ) ;
#5482=DIRECTION ( 'NONE',  ( -0.000000000000000000, -0.000000000000000000, 1.000000000000000000 ) ) ;
#5484=CARTESIAN_POINT ( 'NONE',  ( -29.61203839202723032, -15.40012917324033381, 37.38016955275590192 ) ) ;
#5486=CARTESIAN_POINT ( 'NONE',  ( -4.375757216953428294E-15, -39.50000000000000000, 34.49999999999999289 ) ) ;
#5488=CARTESIAN_POINT ( 'NONE',  ( 24.58208797071834439, 7.298293523701641305, 49.35779847067223614 ) ) ;
#5503=CARTESIAN_POINT ( 'NONE',  ( -23.59115238065502851, -12.85789229732232997, 43.88988317752900770 ) ) ;
#5509=VERTEX_POINT ( 'NONE', #28771 ) ;
#5512=CYLINDRICAL_SURFACE ( 'NONE', #19977, 2.000000000000001776 ) ;
#5526=EDGE_CURVE ( 'NONE', #17814, #5509, #842, .T. ) ;
#5527=VECTOR ( 'NONE', #4856, 1000.000000000000000 ) ;
#5535=CARTESIAN_POINT ( 'NONE',  ( 1.860660329155702231, -42.45830717661258547, 34.61210867867529828 ) ) ;
#5545=CARTESIAN_POINT ( 'NONE',  ( -38.67597152258920801, -5.617507608258466512, 32.13009641412468653 ) ) ;
#5555=CARTESIAN_POINT ( 'NONE',  ( 31.22486525274646496, 15.32888848509420221, 35.97296397489736108 ) ) ;
#5565=FACE_OUTER_BOUND ( 'NONE', #8730, .T. ) ;
#5580=CARTESIAN_POINT ( 'NONE',  ( -33.67377525255856341, -13.97887046878493500, 27.50000000000000000 ) ) ;
#5585=DIRECTION ( 'NONE',  ( 0.000000000000000000, 0.000000000000000000, 1.000000000000000000 ) ) ;
#5594=EDGE_CURVE ( 'NONE', #18416, #3499, #14805, .T. ) ;
#5604=CARTESIAN_POINT ( 'NONE',  ( -12.64130592652783136, 40.29950990793869892, 29.03293690792085258 ) ) ;
#5609=CARTESIAN_POINT ( 'NONE',  ( 34.45795948451156221, -11.47936083950614794, 34.50000000000000000 ) ) ;
#5611=EDGE_LOOP ( 'NONE', ( #13562, #25775, #26393, #14237 ) ) ;
#5613=APPLICATION_CONTEXT ( 'automotive_design' ) ;
#5634=CARTESIAN_POINT ( 'NONE',  ( 31.79271162922634630, -14.90794587988476927, 35.64318943584540733 ) ) ;
#5637=VECTOR ( 'NONE', #10990, 1000.000000000000000 ) ;
#5640=CARTESIAN_POINT ( 'NONE',  ( 23.05503963851395000, 30.35185526021188807, 34.49999999999999289 ) ) ;
#5645=CARTESIAN_POINT ( 'NONE',  ( -24.50428919468314248, -7.442132857256927636, 49.39104690844366274 ) ) ;
#5647=CARTESIAN_POINT ( 'NONE',  ( 23.62400240902267967, -9.724154461249520764, 49.47829057475696146 ) ) ;
#5655=CARTESIAN_POINT ( 'NONE',  ( 14.14241404620503317, 39.63505646587483255, 34.54980534962761141 ) ) ;
#5657=ORIENTED_EDGE ( 'NONE', *, *, #10940, .T. ) ;
#5682=CARTESIAN_POINT ( 'NONE',  ( 33.51208342369034199, -9.877893692955343141, 35.81995677910244780 ) ) ;
#5683=ORIENTED_EDGE ( 'NONE', *, *, #15859, .T. ) ;
#5697=CARTESIAN_POINT ( 'NONE',  ( -25.50709904238008008, -27.59382699987884280, 37.50000000002468425 ) ) ;
#5705=CARTESIAN_POINT ( 'NONE',  ( 32.19782014694307293, 14.25394737442116444, 35.54550565580007770 ) ) ;
#5708=B_SPLINE_CURVE_WITH_KNOTS ( 'NONE', 3,
 ( #30219, #15878, #18673, #20853, #4485, #18835, #20693, #6977, #1988, #4633, #18385, #16488, #6517, #26004 ),
 .UNSPECIFIED., .F., .F.,
 ( 4, 2, 2, 2, 2, 2, 4 ),
 ( 2.108610145906054180E-07, 0.0004867403503157751322, 0.0009732698396169596391, 0.001459799328918144146, 0.001946328818219328653, 0.002919387796821705256, 0.003892446775424082076 ),
 .UNSPECIFIED. ) ;
#5722=CARTESIAN_POINT ( 'NONE',  ( -15.48249060714018199, -35.68301910287905088, 27.50000000000000355 ) ) ;
#5741=EDGE_CURVE ( 'NONE', #13876, #3241, #23121, .T. ) ;
#5742=CARTESIAN_POINT ( 'NONE',  ( 31.70481081259145384, -24.75827009233382725, 30.59596842323437116 ) ) ;
#5748=CARTESIAN_POINT ( 'NONE',  ( -28.23311950821117122, 29.32737283093239711, 30.11920113326423376 ) ) ;
#5757=B_SPLINE_CURVE_WITH_KNOTS ( 'NONE', 3,
 ( #6881, #30736, #18901, #8935, #28107, #19045 ),
 .UNSPECIFIED., .F., .F.,
 ( 4, 2, 4 ),
 ( 0.1293062580255212313, 0.1318912024619483814, 0.1344761468983755315 ),
 .UNSPECIFIED. ) ;
#5763=CARTESIAN_POINT ( 'NONE',  ( -33.42925964089140933, 11.06161099612212695, 39.78814634291943264 ) ) ;
#5767=ORIENTED_EDGE ( 'NONE', *, *, #3632, .T. ) ;
#5779=ORIENTED_EDGE ( 'NONE', *, *, #2346, .T. ) ;
#5786=CARTESIAN_POINT ( 'NONE',  ( 33.53348741818256684, 14.37470038618140933, 34.49999999999998579 ) ) ;
#5790=CARTESIAN_POINT ( 'NONE',  ( 30.50204315964897717, 15.53056155674291539, 40.77182279853379754 ) ) ;
#5792=CARTESIAN_POINT ( 'NONE',  ( 25.18096005886327760, 6.640581704039639988, 48.95928115109020240 ) ) ;
#5794=CIRCLE ( 'NONE', #27214, 36.25735931288072322 ) ;
#5812=CARTESIAN_POINT ( 'NONE',  ( 24.58208797071834439, 7.298293523701643082, 45.11515778355294515 ) ) ;
#5845=CARTESIAN_POINT ( 'NONE',  ( -32.06827542805549314, 14.53851282002520762, 35.54771035678272995 ) ) ;
#5855=FACE_OUTER_BOUND ( 'NONE', #12457, .T. ) ;
#5856=CARTESIAN_POINT ( 'NONE',  ( -38.65970988490578719, -5.757014596993029976, 35.04328188762917051 ) ) ;
#5882=ORIENTED_EDGE ( 'NONE', *, *, #16786, .F. ) ;
#5901=CARTESIAN_POINT ( 'NONE',  ( 36.69132079237465405, -14.42015626554423235, 31.58303039899921316 ) ) ;
#5923=CARTESIAN_POINT ( 'NONE',  ( -24.35970437652574105, 13.37404834226503247, 42.96778633356043287 ) ) ;
#5938=CARTESIAN_POINT ( 'NONE',  ( 29.81954908927654202, -15.48017614753372584, 37.15913391342340333 ) ) ;
#5943=CARTESIAN_POINT ( 'NONE',  ( 33.56327786402390245, 10.34181101807379299, 39.87954049117193023 ) ) ;
#5946=CARTESIAN_POINT ( 'NONE',  ( -35.45878215871336181, -7.046087300371452145, 34.64822579837505856 ) ) ;
#5965=ADVANCED_FACE ( 'NONE', ( #11372 ), #15354, .T. ) ;
#5967=DIRECTION ( 'NONE',  ( -0.000000000000000000, -0.000000000000000000, 1.000000000000000000 ) ) ;
#5970=CARTESIAN_POINT ( 'NONE',  ( -33.52437897089259877, -10.76376600292166863, 35.54771035675473456 ) ) ;
#5971=CARTESIAN_POINT ( 'NONE',  ( -33.51206231511395117, 9.871883628028008673, 40.06435153362845369 ) ) ;
#5974=ORIENTED_EDGE ( 'NONE', *, *, #30325, .T. ) ;
#5995=CARTESIAN_POINT ( 'NONE',  ( -33.03011559203990544, 8.976883822286589876, 36.52918211139306237 ) ) ;
#6008=CARTESIAN_POINT ( 'NONE',  ( -7.885088086771752991, -41.65010312772935208, 28.91342085574027720 ) ) ;
#6027=CARTESIAN_POINT ( 'NONE',  ( 33.36623411648999848, -9.470136927103574465, 40.31594401536676031 ) ) ;
#6044=CARTESIAN_POINT ( 'NONE',  ( -12.81862250463242781, 40.16661589154484346, 29.04586181293521108 ) ) ;
#6053=CARTESIAN_POINT ( 'NONE',  ( -4.776122516674677878E-15, -42.50000000000000000, 28.83974596215560737 ) ) ;
#6099=ORIENTED_EDGE ( 'NONE', *, *, #13186, .F. ) ;
#6102=FACE_OUTER_BOUND ( 'NONE', #18357, .T. ) ;
#6110=CARTESIAN_POINT ( 'NONE',  ( 33.42925964089140933, 11.06161099612213405, 39.78814634291935448 ) ) ;
#6122=CARTESIAN_POINT ( 'NONE',  ( -32.28307784207223108, 8.475829241206282560, 37.38016955275591613 ) ) ;
#6123=EDGE_CURVE ( 'NONE', #29565, #1203, #12131, .T. ) ;
#6139=AXIS2_PLACEMENT_3D ( 'NONE', #7163, #21174, #30698 ) ;
#6143=CARTESIAN_POINT ( 'NONE',  ( -33.43024933835881285, 9.611735609129386404, 35.97296397483977159 ) ) ;
#6144=VERTEX_POINT ( 'NONE', #19601 ) ;
#6146=CARTESIAN_POINT ( 'NONE',  ( -31.79271162922631788, 14.90794587988477815, 35.64318943584552812 ) ) ;
#6162=CARTESIAN_POINT ( 'NONE',  ( -12.34832590236237237, -40.32090071188812885, 34.56244595848355772 ) ) ;
#6164=CARTESIAN_POINT ( 'NONE',  ( -30.03792366816882620, -15.52577997660842435, 41.18702913624207440 ) ) ;
#6168=B_SPLINE_CURVE_WITH_KNOTS ( 'NONE', 3,
 ( #13188, #13345, #18175, #27681, #6310, #29663, #15300, #3466, #10480, #501 ),
 .UNSPECIFIED., .F., .F.,
 ( 4, 2, 2, 2, 4 ),
 ( 0.0007598054600062437158, 0.001542965791078105241, 0.002326126122149966766, 0.003109286453221827857, 0.003892446784293689382 ),
 .UNSPECIFIED. ) ;
#6170=CARTESIAN_POINT ( 'NONE',  ( -24.44496207165490276, 7.595930209050158588, 45.15942333309111945 ) ) ;
#6172=CARTESIAN_POINT ( 'NONE',  ( 23.10264100946039534, 11.84391650453516043, 44.79593483593096437 ) ) ;
#6173=CARTESIAN_POINT ( 'NONE',  ( 31.89119714134807637, 14.79609055705961573, 35.60128781023431799 ) ) ;
#6178=DIRECTION ( 'NONE',  ( 1.000000000000000000, 0.000000000000000000, 0.000000000000000000 ) ) ;
#6182=CARTESIAN_POINT ( 'NONE',  ( 33.41032657756569790, -9.567127522732029377, 40.24698379951695415 ) ) ;
#6200=CARTESIAN_POINT ( 'NONE',  ( -13.58027524052048562, 34.95958275926333414, 37.50000000001884359 ) ) ;
#6207=B_SPLINE_CURVE_WITH_KNOTS ( 'NONE', 3,
 ( #27194, #24382, #22193, #7712 ),
 .UNSPECIFIED., .F., .F.,
 ( 4, 4 ),
 ( 3.018024802580205417E-07, 0.007932103453629116285 ),
 .UNSPECIFIED. ) ;
#6209=CARTESIAN_POINT ( 'NONE',  ( -27.03074382657074537, 6.449748410230984774, 47.21042702067971675 ) ) ;
#6210=CARTESIAN_POINT ( 'NONE',  ( 19.50335127913461974, -36.90537731026830670, 29.35045827479529024 ) ) ;
#6219=CARTESIAN_POINT ( 'NONE',  ( 34.13832859401787090, 12.80067323710188809, 27.50000000000001066 ) ) ;
#6220=ORIENTED_EDGE ( 'NONE', *, *, #4412, .T. ) ;
#6230=DIRECTION ( 'NONE',  ( -0.000000000000000000, -0.000000000000000000, -1.000000000000000000 ) ) ;
#6246=CARTESIAN_POINT ( 'NONE',  ( -36.00000000000000000, 2.601438916704200466, 34.80090346875804386 ) ) ;
#6267=CARTESIAN_POINT ( 'NONE',  ( -33.18396177295070260, 9.163667207889121258, 40.57409041144032358 ) ) ;
#6292=B_SPLINE_CURVE_WITH_KNOTS ( 'NONE', 3,
 ( #15709, #30063, #8703, #25225 ),
 .UNSPECIFIED., .F., .F.,
 ( 4, 4 ),
 ( 3.018024802580205417E-07, 0.007932103453629112816 ),
 .UNSPECIFIED. ) ;
#6300=CARTESIAN_POINT ( 'NONE',  ( 16.58685200597968290, -38.49307988151863213, 29.20042932998627094 ) ) ;
#6310=CARTESIAN_POINT ( 'NONE',  ( -23.36057818983817924, -12.54850586925978284, 48.48255250177239617 ) ) ;
#6316=CARTESIAN_POINT ( 'NONE',  ( -24.44496207165490276, -7.595930209050158588, -16.55003854064094426 ) ) ;
#6344=( NAMED_UNIT ( * ) SI_UNIT ( $, .STERADIAN. ) SOLID_ANGLE_UNIT ( ) );
#6356=CARTESIAN_POINT ( 'NONE',  ( 2.261640607880582632, 42.53980470135267211, 28.83615268921961672 ) ) ;
#6381=CARTESIAN_POINT ( 'NONE',  ( 34.13832859401787090, 12.80067323710188809, 34.80090346875810070 ) ) ;
#6392=CARTESIAN_POINT ( 'NONE',  ( -4.163336342344337027E-14, 1.387778780781445676E-14, 62.49999999999999289 ) ) ;
#6394=CARTESIAN_POINT ( 'NONE',  ( -33.54152001338305666, -10.01313039630840152, 39.99603010802629655 ) ) ;
#6395=EDGE_LOOP ( 'NONE', ( #12597, #22084, #27133, #10403 ) ) ;
#6399=LINE ( 'NONE', #25576, #20887 ) ;
#6416=ORIENTED_EDGE ( 'NONE', *, *, #24246, .T. ) ;
#6428=CARTESIAN_POINT ( 'NONE',  ( 23.94669763007064134, -13.17250946182262972, 47.66948656108987592 ) ) ;
#6429=ORIENTED_EDGE ( 'NONE', *, *, #30719, .T. ) ;
#6446=CARTESIAN_POINT ( 'NONE',  ( -33.42925964089140933, 11.06161099612212695, 35.54550565580014876 ) ) ;
#6454=VECTOR ( 'NONE', #5967, 1000.000000000000000 ) ;
#6465=CARTESIAN_POINT ( 'NONE',  ( 20.12759350631650079, -36.43173182286896150, 29.39766878516364912 ) ) ;
#6472=CARTESIAN_POINT ( 'NONE',  ( -22.65044984052701338, -34.60503960346625263, 29.57823825362870807 ) ) ;
#6475=CARTESIAN_POINT ( 'NONE',  ( -31.89119714134806927, -14.79609055705960863, 39.84392849735367292 ) ) ;
#6492=ORIENTED_EDGE ( 'NONE', *, *, #25807, .F. ) ;
#6507=CARTESIAN_POINT ( 'NONE',  ( -8.682310844383327009, 41.46098991953741120, 34.58670143013237919 ) ) ;
#6513=CARTESIAN_POINT ( 'NONE',  ( -33.42925964089141644, -11.06161099612212695, -16.55003854064094426 ) ) ;
#6517=CARTESIAN_POINT ( 'NONE',  ( 26.81381729043378570, -6.366069288663354087, 43.19821070580849920 ) ) ;
#6521=EDGE_CURVE ( 'NONE', #18778, #438, #603, .T. ) ;
#6527=EDGE_CURVE ( 'NONE', #10056, #18778, #2094, .T. ) ;
#6529=CARTESIAN_POINT ( 'NONE',  ( 32.31576317091161599, -17.59561277345965280, 34.80090346875809360 ) ) ;
#6560=EDGE_LOOP ( 'NONE', ( #6588, #1450, #25113, #17142, #21470, #5154, #22451, #5060, #2308 ) ) ;
#6572=CARTESIAN_POINT ( 'NONE',  ( -23.13350093726293366, 11.03024450687078506, 45.12903505574596608 ) ) ;
#6573=CARTESIAN_POINT ( 'NONE',  ( -19.67362645597749449, 33.08334462853547819, 27.50000000000000000 ) ) ;
#6582=CARTESIAN_POINT ( 'NONE',  ( 27.03074382657074182, -6.449748410230990991, 42.96778633356034049 ) ) ;
#6588=ORIENTED_EDGE ( 'NONE', *, *, #28852, .F. ) ;
#6594=CARTESIAN_POINT ( 'NONE',  ( -32.19782014694307293, 14.25394737442115733, 35.54550565580015586 ) ) ;
#6608=CONICAL_SURFACE ( 'NONE', #24017, 37.50000000000001421, 0.7853981633974500554 ) ;
#6610=CARTESIAN_POINT ( 'NONE',  ( 12.56271066119290936, -40.24229205698606648, 34.56094169196020260 ) ) ;
#6616=EDGE_CURVE ( 'NONE', #23323, #14013, #24083, .T. ) ;
#6620=ORIENTED_EDGE ( 'NONE', *, *, #12282, .T. ) ;
#6621=CARTESIAN_POINT ( 'NONE',  ( -21.56196259436895346, -35.42116262697312123, 29.49711835318369424 ) ) ;
#6656=CARTESIAN_POINT ( 'NONE',  ( -25.53015708495999547, 6.470147010658195086, 44.42018155122911338 ) ) ;
#6672=CARTESIAN_POINT ( 'NONE',  ( 21.86019681245146629, -31.48592878035298170, 27.50000000000001776 ) ) ;
#6680=CARTESIAN_POINT ( 'NONE',  ( -26.11179934312166750, 14.04991663536888957, 45.34931131770228063 ) ) ;
#6681=FACE_OUTER_BOUND ( 'NONE', #9730, .T. ) ;
#6682=EDGE_LOOP ( 'NONE', ( #13034, #27059, #30012, #3163 ) ) ;
#6683=EDGE_CURVE ( 'NONE', #15816, #12560, #22827, .T. ) ;
#6694=ORIENTED_EDGE ( 'NONE', *, *, #15464, .T. ) ;
#6715=LINE ( 'NONE', #1888, #20578 ) ;
#6717=CARTESIAN_POINT ( 'NONE',  ( -30.97476472108959911, 20.16426083678214809, 27.50000000000000711 ) ) ;
#6718=CARTESIAN_POINT ( 'NONE',  ( 34.70577939417261604, -10.49309206032036634, 34.49999999999999289 ) ) ;
#6722=CARTESIAN_POINT ( 'NONE',  ( -35.46011056729421540, 7.038057716383124607, 34.64849135038186745 ) ) ;
#6725=ORIENTED_EDGE ( 'NONE', *, *, #21544, .T. ) ;
#6732=CARTESIAN_POINT ( 'NONE',  ( 8.553213014649442059, -38.39187072122768285, 27.49999999999999645 ) ) ;
#6738=B_SPLINE_CURVE_WITH_KNOTS ( 'NONE', 3,
 ( #19846, #8008, #24671, #979, #10489, #22481, #29520, #8159, #8312, #5812, #15309, #1127 ),
 .UNSPECIFIED., .F., .F.,
 ( 4, 2, 2, 2, 2, 4 ),
 ( 2.975219550396606016E-07, 0.0009689891316535842632, 0.001937680741352128993, 0.002906372351050673722, 0.003390718155899950965, 0.003875063960749227775 ),
 .UNSPECIFIED. ) ;
#6746=LINE ( 'NONE', #1764, #846 ) ;
#6756=CARTESIAN_POINT ( 'NONE',  ( 29.13062620811776782, -28.39040064518643547, 30.21738835640542220 ) ) ;
#6767=CARTESIAN_POINT ( 'NONE',  ( 4.216636297896259045, 37.26217892624188011, 37.50000000000000000 ) ) ;
#6776=EDGE_CURVE ( 'NONE', #19006, #4914, #19706, .T. ) ;
#6785=CARTESIAN_POINT ( 'NONE',  ( 32.28307784207223108, -8.475829241206289666, 37.38016955275583086 ) ) ;
#6788=ORIENTED_EDGE ( 'NONE', *, *, #22724, .T. ) ;
#6797=VERTEX_POINT ( 'NONE', #16267 ) ;
#6803=CARTESIAN_POINT ( 'NONE',  ( -38.62541652119597302, 5.911948292485620371, 32.11511063132802235 ) ) ;
#6805=DIRECTION ( 'NONE',  ( 0.3598999890241668664, 0.9329908884337534403, 0.000000000000000000 ) ) ;
#6808=ORIENTED_EDGE ( 'NONE', *, *, #14327, .T. ) ;
#6812=CARTESIAN_POINT ( 'NONE',  ( -4.163336342344337027E-14, 1.387778780781445676E-14, 35.37867965644034740 ) ) ;
#6825=ORIENTED_EDGE ( 'NONE', *, *, #2163, .T. ) ;
#6843=ADVANCED_FACE ( 'NONE', ( #4415 ), #18928, .F. ) ;
#6856=CARTESIAN_POINT ( 'NONE',  ( 11.43275458328725591, -37.45803590232208080, 34.49999999999998579 ) ) ;
#6861=ORIENTED_EDGE ( 'NONE', *, *, #16607, .F. ) ;
#6868=CARTESIAN_POINT ( 'NONE',  ( -32.32764558496669594, 17.38770747897534719, 27.50000000000000000 ) ) ;
#6881=CARTESIAN_POINT ( 'NONE',  ( -4.776122516674677878E-15, -42.50000000000000000, 28.83974596215560737 ) ) ;
#6885=CARTESIAN_POINT ( 'NONE',  ( 18.66785090198818864, 33.79720267974621351, 27.50000000000000000 ) ) ;
#6917=CARTESIAN_POINT ( 'NONE',  ( 20.93653161406057350, -35.88774558615511978, 34.51026993352196115 ) ) ;
#6923=B_SPLINE_CURVE_WITH_KNOTS ( 'NONE', 3,
 ( #14990, #24502, #24657, #10313, #3147, #12670, #22164, #19829, #29352, #17496, #5645, #3292 ),
 .UNSPECIFIED., .F., .F.,
 ( 4, 2, 2, 2, 2, 4 ),
 ( 2.975219550396606016E-07, 0.0009689891316535838295, 0.001937680741352128125, 0.002906372351050672421, 0.003390718155899948363, 0.003875063960749225173 ),
 .UNSPECIFIED. ) ;
#6944=FACE_OUTER_BOUND ( 'NONE', #6395, .T. ) ;
#6951=CARTESIAN_POINT ( 'NONE',  ( 32.44949699048088121, -8.540025205420070264, 37.20290368958222160 ) ) ;
#6955=DIRECTION ( 'NONE',  ( -0.000000000000000000, -0.000000000000000000, -1.000000000000000000 ) ) ;
#6969=CARTESIAN_POINT ( 'NONE',  ( -17.79898064049163153, 37.82295783581751891, 29.26401803458472628 ) ) ;
#6971=CARTESIAN_POINT ( 'NONE',  ( 27.86235613436987890, -14.72519157938688927, 43.48653168448677064 ) ) ;
#6977=CARTESIAN_POINT ( 'NONE',  ( 25.41307773079511634, -6.523700759042267983, 44.52046879171659555 ) ) ;
#7015=CARTESIAN_POINT ( 'NONE',  ( 15.62938862465957079, -35.64705970074183483, 34.49999999999999289 ) ) ;
#7039=CARTESIAN_POINT ( 'NONE',  ( 33.69370807471729989, -13.92103290742843491, 27.50000000000000355 ) ) ;
#7063=CARTESIAN_POINT ( 'NONE',  ( 37.08686162832535871, 13.21332193651624110, 31.68138836149219628 ) ) ;
#7076=VECTOR ( 'NONE', #30306, 1000.000000000000000 ) ;
#7088=EDGE_CURVE ( 'NONE', #18831, #26574, #6715, .T. ) ;
#7091=DIRECTION ( 'NONE',  ( 1.000000000000000000, 0.000000000000000000, 0.000000000000000000 ) ) ;
#7117=EDGE_CURVE ( 'NONE', #27891, #12561, #1669, .T. ) ;
#7120=CARTESIAN_POINT ( 'NONE',  ( -23.38069191132970204, 29.32513219524850001, 37.49999999996538236 ) ) ;
#7132=CARTESIAN_POINT ( 'NONE',  ( -23.07950435457351190, 11.50806656539842798, 49.21048435262080289 ) ) ;
#7134=B_SPLINE_CURVE_WITH_KNOTS ( 'NONE', 3,
 ( #4903, #14421, #11615, #14093 ),
 .UNSPECIFIED., .F., .F.,
 ( 4, 4 ),
 ( 3.022186913359086288E-07, 0.007932103869840195776 ),
 .UNSPECIFIED. ) ;
#7155=CARTESIAN_POINT ( 'NONE',  ( -26.12047388987420149, 6.311255530320346807, 48.12792051007069460 ) ) ;
#7163=CARTESIAN_POINT ( 'NONE',  ( 0.000000000000000000, 0.000000000000000000, 34.49999999999999289 ) ) ;
#7167=CARTESIAN_POINT ( 'NONE',  ( -23.36055057548231062, 12.54866584153426601, 48.48250221505454505 ) ) ;
#7172=FACE_OUTER_BOUND ( 'NONE', #27412, .T. ) ;
#7181=CARTESIAN_POINT ( 'NONE',  ( -22.64188265567332436, -30.81688647342193121, 27.50000000000000711 ) ) ;
#7185=CARTESIAN_POINT ( 'NONE',  ( -2.048514414209405832, -39.45186992530642556, 34.50000000000000711 ) ) ;
#7194=CARTESIAN_POINT ( 'NONE',  ( 3.101722653984818834, 39.35894504374194014, 27.49999999999999645 ) ) ;
#7210=CARTESIAN_POINT ( 'NONE',  ( -33.56615453960540663, 10.45399542313511354, 35.60128781019762556 ) ) ;
#7213=CARTESIAN_POINT ( 'NONE',  ( 25.41822862649771508, 27.59854655694143588, 37.49999999990964028 ) ) ;
#7266=CARTESIAN_POINT ( 'NONE',  ( -37.98255541114690459, 9.730631687238020078, 31.92508531691350981 ) ) ;
#7279=EDGE_CURVE ( 'NONE', #17105, #13217, #15621, .T. ) ;
#7302=DIRECTION ( 'NONE',  ( 1.000000000000000000, 0.000000000000000000, 0.000000000000000000 ) ) ;
#7309=( BOUNDED_SURFACE ( )  B_SPLINE_SURFACE ( 3, 2, ( 
 ( #15183, #25168, #29703 ),
 ( #22667, #17392, #26914 ),
 ( #8515, #8347, #27527 ),
 ( #3347, #3812, #13335 ),
 ( #17543, #22832, #19719 ),
 ( #12879, #5535, #15035 ),
 ( #27062, #24550, #10374 ),
 ( #24705, #22378, #10522 ),
 ( #2070, #20642, #20936 ),
 ( #18620, #20494, #25643 ),
 ( #9103, #6610, #25938 ),
 ( #4259, #4570, #16125 ),
 ( #4420, #27980, #28291 ),
 ( #6300, #13787, #14073 ),
 ( #18772, #27672, #30607 ),
 ( #6465, #25333, #23284 ),
 ( #13494, #6917, #8794 ),
 ( #16427, #15813, #15973 ),
 ( #28132, #30460, #30314 ),
 ( #3974, #1926, #11451 ),
 ( #6756, #16271, #25794 ),
 ( #13935, #23432, #22978 ),
 ( #11145, #11593, #11293 ),
 ( #8961, #13648, #21087 ),
 ( #1483, #1634, #9253 ),
 ( #10995, #30161, #30015 ),
 ( #8656, #18320, #18164 ),
 ( #27836, #25493, #4118 ),
 ( #20789, #23130, #1775 ),
 ( #18476, #19215, #21552 ),
 ( #29049, #14394, #23735 ),
 ( #12369, #26709, #30770 ),
 ( #21238, #18933, #7536 ),
 ( #2847, #9868, #23901 ),
 ( #19069, #5188, #9416 ),
 ( #24194, #14690, #2692 ),
 ( #28438, #16727, #14548 ),
 ( #2544, #21405, #12203 ),
 ( #7063, #26239, #21871 ),
 ( #12060, #47, #19383 ),
 ( #28588, #9557, #28901 ),
 ( #26561, #505, #11914 ),
 ( #7690, #17037, #11744 ),
 ( #2387, #344, #28744 ),
 ( #7382, #4878, #10025 ),
 ( #21703, #19534, #14222 ),
 ( #16571, #26088, #17189 ),
 ( #5338, #23582, #7213 ),
 ( #188, #9705, #4720 ),
 ( #2225, #16890, #26409 ),
 ( #5035, #24046, #19678 ),
 ( #1285, #12836, #10640 ),
 ( #15150, #3620, #29366 ),
 ( #8307, #17507, #8005 ),
 ( #27027, #20150, #24837 ),
 ( #26876, #22338, #1125 ),
 ( #14849, #5655, #10171 ),
 ( #24669, #3473, #19997 ),
 ( #976, #29668, #17824 ),
 ( #3307, #29200, #10486 ) ),
 .UNSPECIFIED., .F., .F., .T. ) 
 B_SPLINE_SURFACE_WITH_KNOTS ( ( 4, 2, 2, 2, 2, 2, 2, 2, 2, 2, 2, 2, 2, 2, 2, 2, 2, 2, 2, 2, 2, 2, 2, 2, 2, 2, 2, 2, 2, 4 ),
 ( 3, 3 ),
 ( 0.09646856835573283662, 0.09948321111685021201, 0.1009905324974089136, 0.1024978538779676013, 0.1085271394002023659, 0.1100344607807610675, 0.1115417821613197552, 0.1145564249224371445, 0.1175710676835545199, 0.1205857104446719091, 0.1266149959669066738, 0.1326442814891414523, 0.1356589242502588277, 0.1386735670113762309, 0.1447028525336109817, 0.1477174952947283570, 0.1492248166752870309, 0.1507321380558457324, 0.1567614235780805110, 0.1597760663391978864, 0.1627907091003152895, 0.1688199946225500403, 0.1703273160031087419, 0.1718346373836674157, 0.1748492801447847911, 0.1808785656670195696, 0.1823858870475782434, 0.1838932084281369450, 0.1869078511892543482, 0.1929371367114890989 ),
 ( 0.000000000000000000, 1.000000000000000000 ),
 .UNSPECIFIED. ) 
 GEOMETRIC_REPRESENTATION_ITEM ( )  RATIONAL_B_SPLINE_SURFACE ( (
 ( 1.000000000000000000, 0.8675417673879289859, 1.000000000000000000),
 ( 1.000000000000000000, 0.8667209715531846159, 1.000000000000000000),
 ( 1.000000000000000000, 0.8662263239862698638, 1.000000000000000000),
 ( 1.000000000000000000, 0.8659995305180094860, 1.000000000000000000),
 ( 1.000000000000000000, 0.8660104782249490318, 1.000000000000000000),
 ( 1.000000000000000000, 0.8662041757988804269, 1.000000000000000000),
 ( 1.000000000000000000, 0.8663863992244035250, 1.000000000000000000),
 ( 1.000000000000000000, 0.8677117148204597230, 1.000000000000000000),
 ( 1.000000000000000000, 0.8700966207775098216, 1.000000000000000000),
 ( 1.000000000000000000, 0.8745420513867560031, 1.000000000000000000),
 ( 1.000000000000000000, 0.8755007923160716965, 1.000000000000000000),
 ( 1.000000000000000000, 0.8775326389012688688, 1.000000000000000000),
 ( 1.000000000000000000, 0.8786077117299072592, 1.000000000000000000),
 ( 1.000000000000000000, 0.8819935310329167777, 1.000000000000000000),
 ( 1.000000000000000000, 0.8844646895995935676, 1.000000000000000000),
 ( 1.000000000000000000, 0.8897514236679686661, 1.000000000000000000),
 ( 1.000000000000000000, 0.8925717272467494912, 1.000000000000000000),
 ( 1.000000000000000000, 0.8984586818434432409, 1.000000000000000000),
 ( 1.000000000000000000, 0.9014857458774653276, 1.000000000000000000),
 ( 1.000000000000000000, 0.9106811941533423660, 1.000000000000000000),
 ( 1.000000000000000000, 0.9169643886478042738, 1.000000000000000000),
 ( 1.000000000000000000, 0.9291626511573400915, 1.000000000000000000),
 ( 1.000000000000000000, 0.9349057736410160135, 1.000000000000000000),
 ( 1.000000000000000000, 0.9425642407771720466, 1.000000000000000000),
 ( 1.000000000000000000, 0.9449584557358955417, 1.000000000000000000),
 ( 1.000000000000000000, 0.9493596902480637700, 1.000000000000000000),
 ( 1.000000000000000000, 0.9513682277052729619, 1.000000000000000000),
 ( 1.000000000000000000, 0.9566191346130005213, 1.000000000000000000),
 ( 1.000000000000000000, 0.9591281150650757814, 1.000000000000000000),
 ( 1.000000000000000000, 0.9612060428348171426, 1.000000000000000000),
 ( 1.000000000000000000, 0.9616180368580454774, 1.000000000000000000),
 ( 1.000000000000000000, 0.9617930603854571991, 1.000000000000000000),
 ( 1.000000000000000000, 0.9617771003161980081, 1.000000000000000000),
 ( 1.000000000000000000, 0.9615975401732786976, 1.000000000000000000),
 ( 1.000000000000000000, 0.9614342877366656159, 1.000000000000000000),
 ( 1.000000000000000000, 0.9602599180209367979, 1.000000000000000000),
 ( 1.000000000000000000, 0.9581730223097011390, 1.000000000000000000),
 ( 1.000000000000000000, 0.9535175983937561606, 1.000000000000000000),
 ( 1.000000000000000000, 0.9517118983112912156, 1.000000000000000000),
 ( 1.000000000000000000, 0.9476286036465969564, 1.000000000000000000),
 ( 1.000000000000000000, 0.9453763728113453446, 1.000000000000000000),
 ( 1.000000000000000000, 0.9381189311205525572, 1.000000000000000000),
 ( 1.000000000000000000, 0.9326041533762798874, 1.000000000000000000),
 ( 1.000000000000000000, 0.9252136989611822182, 1.000000000000000000),
 ( 1.000000000000000000, 0.9237107470788312735, 1.000000000000000000),
 ( 1.000000000000000000, 0.9206640173840989760, 1.000000000000000000),
 ( 1.000000000000000000, 0.9191158710780323871, 1.000000000000000000),
 ( 1.000000000000000000, 0.9144587407289394010, 1.000000000000000000),
 ( 1.000000000000000000, 0.9113459265957564170, 1.000000000000000000),
 ( 1.000000000000000000, 0.9021094256030967040, 1.000000000000000000),
 ( 1.000000000000000000, 0.8960840667680185501, 1.000000000000000000),
 ( 1.000000000000000000, 0.8891528055769346572, 1.000000000000000000),
 ( 1.000000000000000000, 0.8877968478283493337, 1.000000000000000000),
 ( 1.000000000000000000, 0.8851579642536796522, 1.000000000000000000),
 ( 1.000000000000000000, 0.8838757127171860128, 1.000000000000000000),
 ( 1.000000000000000000, 0.8802090789781089608, 1.000000000000000000),
 ( 1.000000000000000000, 0.8779855326665648718, 1.000000000000000000),
 ( 1.000000000000000000, 0.8720740473562953454, 1.000000000000000000),
 ( 1.000000000000000000, 0.8691432809519210601, 1.000000000000000000),
 ( 1.000000000000000000, 0.8675023601337629175, 1.000000000000000000) ) ) 
 REPRESENTATION_ITEM ( '' )  SURFACE ( )  );
#7342=CARTESIAN_POINT ( 'NONE',  ( -36.00052790658070023, 0.5797355074648735673, 27.50000000000000711 ) ) ;
#7366=LINE ( 'NONE', #16407, #11347 ) ;
#7382=CARTESIAN_POINT ( 'NONE',  ( 30.84961167908536339, 26.01027997894835764, 30.46573359564818162 ) ) ;
#7387=CARTESIAN_POINT ( 'NONE',  ( 30.53339558441486190, -7.800891647352842462, 39.24389099736750097 ) ) ;
#7396=AXIS2_PLACEMENT_3D ( 'NONE', #9486, #28514, #21014 ) ;
#7403=CARTESIAN_POINT ( 'NONE',  ( -23.16720440049831709, -10.90834004837188154, 45.15082199682045427 ) ) ;
#7430=AXIS2_PLACEMENT_3D ( 'NONE', #12288, #22093, #5110 ) ;
#7432=CARTESIAN_POINT ( 'NONE',  ( -32.89458440824127194, 18.04996087680839167, 37.50000000007908341 ) ) ;
#7455=VERTEX_POINT ( 'NONE', #5763 ) ;
#7462=DIRECTION ( 'NONE',  ( 0.000000000000000000, 0.000000000000000000, 1.000000000000000000 ) ) ;
#7477=CARTESIAN_POINT ( 'NONE',  ( 38.96677131950519879, -1.867903411460851926, 32.22156839220826896 ) ) ;
#7486=VERTEX_POINT ( 'NONE', #5923 ) ;
#7502=CARTESIAN_POINT ( 'NONE',  ( -23.21352257770656990, 10.78826658734919519, 49.40206402021039622 ) ) ;
#7522=CARTESIAN_POINT ( 'NONE',  ( 33.42925964089140933, 11.06161099612213405, 39.78814634291935448 ) ) ;
#7533=EDGE_CURVE ( 'NONE', #28104, #2857, #4756, .T. ) ;
#7536=CARTESIAN_POINT ( 'NONE',  ( 37.50184436008131428, 0.5407290483799589431, 37.50000000002315659 ) ) ;
#7542=DIRECTION ( 'NONE',  ( -0.000000000000000000, -0.000000000000000000, 1.000000000000000000 ) ) ;
#7548=ORIENTED_EDGE ( 'NONE', *, *, #12678, .T. ) ;
#7550=CARTESIAN_POINT ( 'NONE',  ( -23.21352257770656990, 10.78826658734919519, 49.40206402021039622 ) ) ;
#7555=CARTESIAN_POINT ( 'NONE',  ( 26.11179934312166395, 14.04991663536889490, 45.34931131770220247 ) ) ;
#7579=DIRECTION ( 'NONE',  ( 1.000000000000000000, 0.000000000000000000, 0.000000000000000000 ) ) ;
#7581=VERTEX_POINT ( 'NONE', #28481 ) ;
#7582=CARTESIAN_POINT ( 'NONE',  ( 34.70577939417254498, 10.49309206032065944, 34.49999999999999289 ) ) ;
#7586=CARTESIAN_POINT ( 'NONE',  ( -37.98447197189175739, -9.661085588429401128, 34.97777146685444905 ) ) ;
#7588=CARTESIAN_POINT ( 'NONE',  ( 24.03448224033878944, 8.660042335149841009, 45.23564988763769179 ) ) ;
#7596=CARTESIAN_POINT ( 'NONE',  ( 22.49999999999992184, 1.663324310589599759E-14, 62.49999999999999289 ) ) ;
#7609=AXIS2_PLACEMENT_3D ( 'NONE', #4721, #21553, #21239 ) ;
#7617=ORIENTED_EDGE ( 'NONE', *, *, #25695, .F. ) ;
#7626=CARTESIAN_POINT ( 'NONE',  ( -33.37350925571147542, 22.02919766087737941, 30.87635845694642711 ) ) ;
#7639=CARTESIAN_POINT ( 'NONE',  ( 32.19782014694307293, 14.25394737442116444, 35.54550565580007770 ) ) ;
#7650=CARTESIAN_POINT ( 'NONE',  ( -21.55879915780394285, -31.64813929209768517, 34.49999999999999289 ) ) ;
#7666=LINE ( 'NONE', #14672, #8856 ) ;
#7670=CARTESIAN_POINT ( 'NONE',  ( 32.19782014694307293, 14.25394737442116444, 39.78814634291936159 ) ) ;
#7690=CARTESIAN_POINT ( 'NONE',  ( 33.03869540315597675, 22.74296903121848956, 30.80490156986919814 ) ) ;
#7692=B_SPLINE_CURVE_WITH_KNOTS ( 'NONE', 3,
 ( #1890, #3943, #6428, #25749, #30125, #23401, #30430, #27800, #15943, #8927, #25457, #11417 ),
 .UNSPECIFIED., .F., .F.,
 ( 4, 2, 2, 2, 2, 4 ),
 ( 2.975096543230397156E-07, 0.0009689891193463220660, 0.001937680729038321250, 0.002906372338730320217, 0.003390718143576314497, 0.003875063948422308776 ),
 .UNSPECIFIED. ) ;
#7708=CARTESIAN_POINT ( 'NONE',  ( -34.17816363167221994, 12.44541626675085588, 34.50000000000000711 ) ) ;
#7712=CARTESIAN_POINT ( 'NONE',  ( -32.28307784207223108, 8.475829241206282560, 37.38016955275591613 ) ) ;
#7738=CARTESIAN_POINT ( 'NONE',  ( -23.62400240902268322, -9.724154461249517212, 45.23564988763774863 ) ) ;
#7741=CARTESIAN_POINT ( 'NONE',  ( -28.19317390287710623, -29.49677466076099819, 34.53603776002483272 ) ) ;
#7757=DIRECTION ( 'NONE',  ( 1.000000000000000000, 0.000000000000000000, 0.000000000000000000 ) ) ;
#7761=DIRECTION ( 'NONE',  ( 1.000000000000000000, 0.000000000000000000, 0.000000000000000000 ) ) ;
#7774=CARTESIAN_POINT ( 'NONE',  ( 19.67838142173201987, 33.09896098428890809, 27.50000000000000000 ) ) ;
#7776=CARTESIAN_POINT ( 'NONE',  ( 36.86322900007326808, 13.93456307833209706, 31.62480519666989309 ) ) ;
#7781=CARTESIAN_POINT ( 'NONE',  ( -36.50611713474064146, -15.17355836286742843, 31.53147891484856657 ) ) ;
#7799=CARTESIAN_POINT ( 'NONE',  ( -6.606788361478927563, -38.83273613297759397, 34.49999999999999289 ) ) ;
#7800=CARTESIAN_POINT ( 'NONE',  ( -35.97269501643903311, 1.773469557544170572, 34.75180443448076062 ) ) ;
#7812=ORIENTED_EDGE ( 'NONE', *, *, #28636, .F. ) ;
#7818=CARTESIAN_POINT ( 'NONE',  ( 33.17909676736307034, 15.33239136497788913, 34.49999999999997868 ) ) ;
#7838=CYLINDRICAL_SURFACE ( 'NONE', #17022, 1.999999999999998224 ) ;
#7847=ORIENTED_EDGE ( 'NONE', *, *, #10125, .F. ) ;
#7852=ORIENTED_EDGE ( 'NONE', *, *, #2103, .T. ) ;
#7856=CARTESIAN_POINT ( 'NONE',  ( -23.07950435457351190, 11.50806656539842798, 49.21048435262080289 ) ) ;
#7858=CARTESIAN_POINT ( 'NONE',  ( -4.163336342344337027E-14, 1.387778780781445676E-14, 62.49999999999999289 ) ) ;
#7880=ORIENTED_EDGE ( 'NONE', *, *, #25501, .F. ) ;
#7885=FACE_OUTER_BOUND ( 'NONE', #25076, .T. ) ;
#7889=CARTESIAN_POINT ( 'NONE',  ( -4.163336342344337027E-14, 1.387778780781445676E-14, 37.50000000000000000 ) ) ;
#7901=CARTESIAN_POINT ( 'NONE',  ( -38.35800364550046027, -7.710258930485773377, 35.01326192470217080 ) ) ;
#7943=AXIS2_PLACEMENT_3D ( 'NONE', #7889, #17081, #7579 ) ;
#7946=CARTESIAN_POINT ( 'NONE',  ( 37.92610032463591807, 10.23617371602907689, 31.90285370532496856 ) ) ;
#7951=CARTESIAN_POINT ( 'NONE',  ( -37.86918475753925861, -10.24225134995086073, 31.89299558116904265 ) ) ;
#7961=CARTESIAN_POINT ( 'NONE',  ( 23.21352257770656635, -10.78826658734920052, 45.15942333309103418 ) ) ;
#7971=ORIENTED_EDGE ( 'NONE', *, *, #28194, .T. ) ;
#7988=CARTESIAN_POINT ( 'NONE',  ( 27.86772728142310740, 25.09083747725281555, 34.49999999999999289 ) ) ;
#8005=CARTESIAN_POINT ( 'NONE',  ( 15.48300807700231019, 34.15967020736680837, 37.50000000001828937 ) ) ;
#8008=CARTESIAN_POINT ( 'NONE',  ( 26.81368379037234817, 6.366017791192970066, 43.19835251265425313 ) ) ;
#8018=CARTESIAN_POINT ( 'NONE',  ( -23.81715554101158006, 29.69269061775747787, 34.50000000000000000 ) ) ;
#8022=ORIENTED_EDGE ( 'NONE', *, *, #21930, .T. ) ;
#8024=CARTESIAN_POINT ( 'NONE',  ( -24.35970437652574105, -13.37404834226503070, 42.96778633356041865 ) ) ;
#8035=CARTESIAN_POINT ( 'NONE',  ( -33.01877980957529957, -12.12572312222180315, 35.60092001944731521 ) ) ;
#8047=ADVANCED_FACE ( 'NONE', ( #13937 ), #25644, .T. ) ;
#8051=CARTESIAN_POINT ( 'NONE',  ( -37.53333450813131833, 2.083350403252341998, 37.49999999994167865 ) ) ;
#8063=CARTESIAN_POINT ( 'NONE',  ( -32.19782014694307293, 14.25394737442115733, 35.54550565580015586 ) ) ;
#8067=ORIENTED_EDGE ( 'NONE', *, *, #15231, .F. ) ;
#8083=ORIENTED_EDGE ( 'NONE', *, *, #26013, .T. ) ;
#8100=CARTESIAN_POINT ( 'NONE',  ( -10.21480246439553063, 41.11241556754047366, 28.96073186326400872 ) ) ;
#8101=CARTESIAN_POINT ( 'NONE',  ( 77.99999999999998579, -42.50000000000002132, 32.26246401786215756 ) ) ;
#8115=VERTEX_POINT ( 'NONE', #5339 ) ;
#8128=CARTESIAN_POINT ( 'NONE',  ( -32.19782014694307293, 14.25394737442115733, 39.78814634291943975 ) ) ;
#8137=CARTESIAN_POINT ( 'NONE',  ( -15.85884089648730999, 35.55173462727350397, 27.50000000000000355 ) ) ;
#8141=CARTESIAN_POINT ( 'NONE',  ( 24.50428919468314959, 7.442132857256931189, 49.39104690844359880 ) ) ;
#8144=CARTESIAN_POINT ( 'NONE',  ( 33.56327786402390245, 10.46063060613185414, 35.60191137445556819 ) ) ;
#8145=CARTESIAN_POINT ( 'NONE',  ( -23.07950435457403415, 11.62838985844543060, 44.91415175113220215 ) ) ;
#8158=ORIENTED_EDGE ( 'NONE', *, *, #7088, .T. ) ;
#8159=CARTESIAN_POINT ( 'NONE',  ( 24.86084284002701850, 6.930828199065646622, 44.94877300773885764 ) ) ;
#8196=CARTESIAN_POINT ( 'NONE',  ( -36.72813896306210069, -7.597066778515316088, 37.50000000000667200 ) ) ;
#8200=FACE_OUTER_BOUND ( 'NONE', #9264, .T. ) ;
#8236=ADVANCED_FACE ( 'NONE', ( #506 ), #7838, .F. ) ;
#8247=CARTESIAN_POINT ( 'NONE',  ( -4.163336342344337027E-14, 1.387778780781445676E-14, 34.49999999999999289 ) ) ;
#8249=CARTESIAN_POINT ( 'NONE',  ( -33.30753377797442027, -22.11854778782412367, 30.86655168617016187 ) ) ;
#8258=VERTEX_POINT ( 'NONE', #289 ) ;
#8270=MECHANICAL_DESIGN_GEOMETRIC_PRESENTATION_REPRESENTATION('',(#27682),#21193);
#8279=CARTESIAN_POINT ( 'NONE',  ( 32.06827542805550024, -14.53851282002520229, 35.54771035678264468 ) ) ;
#8285=CARTESIAN_POINT ( 'NONE',  ( 32.44940373544195467, 8.539989232413363496, 41.44564370983190571 ) ) ;
#8288=CARTESIAN_POINT ( 'NONE',  ( -21.86019681245148405, 31.48592878035298170, 34.80090346875805807 ) ) ;
#8307=CARTESIAN_POINT ( 'NONE',  ( 18.08806846220652531, 37.65969142884505771, 29.27956356433786311 ) ) ;
#8312=CARTESIAN_POINT ( 'NONE',  ( 24.75988009833579540, 7.043597625963923470, 45.01551998635105889 ) ) ;
#8314=CARTESIAN_POINT ( 'NONE',  ( -32.94612346989018192, 8.892333671926630601, 40.87496192031042597 ) ) ;
#8347=CARTESIAN_POINT ( 'NONE',  ( -2.296078483958558625, -42.45314922741754771, 34.61196682005081726 ) ) ;
#8363=CARTESIAN_POINT ( 'NONE',  ( 32.19782014694308003, -14.25394737442115201, 39.78814634291934738 ) ) ;
#8395=CARTESIAN_POINT ( 'NONE',  ( -22.50000000000000711, 1.020384741037239916E-14, 52.50000000000000000 ) ) ;
#8399=CARTESIAN_POINT ( 'NONE',  ( -5.078594737417330585, 37.17323350146568828, 37.50000000004207834 ) ) ;
#8403=CARTESIAN_POINT ( 'NONE',  ( 24.44496207165490276, 7.595930209050162141, 45.15942333309104129 ) ) ;
#8421=CARTESIAN_POINT ( 'NONE',  ( 31.18890335284659443, -19.89223002944918761, 34.80090346875810781 ) ) ;
#8427=EDGE_CURVE ( 'NONE', #4181, #18831, #29711, .T. ) ;
#8435=CARTESIAN_POINT ( 'NONE',  ( 23.21076833940160000, 12.23288291591659771, 48.76310947893255587 ) ) ;
#8438=ADVANCED_FACE ( 'NONE', ( #14642 ), #2793, .F. ) ;
#8453=ORIENTED_EDGE ( 'NONE', *, *, #3632, .F. ) ;
#8456=CARTESIAN_POINT ( 'NONE',  ( 33.03707461445869598, 8.975870916883787132, 40.76550527633506960 ) ) ;
#8459=CARTESIAN_POINT ( 'NONE',  ( -21.86019681245147694, -31.48592878035298170, 27.50000000000000355 ) ) ;
#8477=CARTESIAN_POINT ( 'NONE',  ( -4.776122516674677878E-15, -42.50000000000000000, 27.50000000000000355 ) ) ;
#8515=CARTESIAN_POINT ( 'NONE',  ( -2.341318239117458511, -42.45126916401905959, 28.84393386495551681 ) ) ;
#8524=CARTESIAN_POINT ( 'NONE',  ( -20.69299247485714588, -36.03354106283070024, 34.51170679603197300 ) ) ;
#8533=DIRECTION ( 'NONE',  ( 0.000000000000000000, 0.000000000000000000, 1.000000000000000000 ) ) ;
#8535=CARTESIAN_POINT ( 'NONE',  ( -24.35970437652574105, -13.37404834226503070, -16.55003854064094426 ) ) ;
#8574=CARTESIAN_POINT ( 'NONE',  ( 23.69412710310942316, 29.84645176427128277, 34.80090346875809360 ) ) ;
#8588=CARTESIAN_POINT ( 'NONE',  ( -33.03705654931147251, -8.970011997839668183, 40.76699977217946724 ) ) ;
#8596=CARTESIAN_POINT ( 'NONE',  ( 33.21383100183306425, 9.208170138131603011, 40.53341495146639772 ) ) ;
#8599=CARTESIAN_POINT ( 'NONE',  ( -9.268856789657290207, -38.25380398711768493, 34.80090346875804386 ) ) ;
#8616=LINE ( 'NONE', #18127, #30836 ) ;
#8618=CARTESIAN_POINT ( 'NONE',  ( -33.54152001338305666, -10.01313039630840152, 35.75338942090700556 ) ) ;
#8631=EDGE_CURVE ( 'NONE', #11387, #30416, #21311, .T. ) ;
#8656=CARTESIAN_POINT ( 'NONE',  ( 37.01788418253418200, -13.43971458426429066, 31.66419126466463752 ) ) ;
#8667=CARTESIAN_POINT ( 'NONE',  ( -30.38302862529102200, -15.53680216053817986, 40.87496192038616982 ) ) ;
#8699=CARTESIAN_POINT ( 'NONE',  ( 4.963855673496207821, 42.15448181593355059, 34.60401223484481648 ) ) ;
#8703=CARTESIAN_POINT ( 'NONE',  ( 30.53339558441486190, -7.800891647352842462, 43.48653168448678485 ) ) ;
#8708=CARTESIAN_POINT ( 'NONE',  ( 5.139473829620250456, -42.22092639811037174, 28.86348903593575699 ) ) ;
#8716=CARTESIAN_POINT ( 'NONE',  ( 34.83396020575241891, -10.30249279383517624, 34.80090346875810070 ) ) ;
#8721=CARTESIAN_POINT ( 'NONE',  ( 33.42925964089141644, -11.06161099612213228, 35.54550565580004928 ) ) ;
#8726=CYLINDRICAL_SURFACE ( 'NONE', #12936, 2.000000000000001776 ) ;
#8730=EDGE_LOOP ( 'NONE', ( #18214, #27262, #21690, #8158, #1948 ) ) ;
#8736=CARTESIAN_POINT ( 'NONE',  ( 32.28307784207223108, -8.475829241206289666, 41.62281023987511475 ) ) ;
#8739=CARTESIAN_POINT ( 'NONE',  ( -36.00000000000000000, -2.601438916704193360, 34.80090346875805096 ) ) ;
#8794=CARTESIAN_POINT ( 'NONE',  ( 18.39838276040765308, -32.69867910685736234, 37.50000000001998757 ) ) ;
#8797=ORIENTED_EDGE ( 'NONE', *, *, #30719, .F. ) ;
#8807=CARTESIAN_POINT ( 'NONE',  ( -19.72128910681292169, -31.90111139983629229, 37.50000000003792167 ) ) ;
#8809=CARTESIAN_POINT ( 'NONE',  ( -32.06725342158289038, -14.54034564589948708, 39.79052675593695199 ) ) ;
#8817=CARTESIAN_POINT ( 'NONE',  ( 23.21352257770656990, 10.78826658734920230, 45.15942333309104129 ) ) ;
#8823=AXIS2_PLACEMENT_3D ( 'NONE', #2643, #4824, #4675 ) ;
#8827=LINE ( 'NONE', #8535, #26481 ) ;
#8831=ORIENTED_EDGE ( 'NONE', *, *, #13390, .F. ) ;
#8856=VECTOR ( 'NONE', #5482, 1000.000000000000000 ) ;
#8858=FACE_OUTER_BOUND ( 'NONE', #18944, .T. ) ;
#8862=VECTOR ( 'NONE', #29457, 1000.000000000000000 ) ;
#8867=CARTESIAN_POINT ( 'NONE',  ( 25.53015708495999547, -6.470147010658199527, 48.66282223834831200 ) ) ;
#8878=CARTESIAN_POINT ( 'NONE',  ( 36.00000000000001421, 2.601438916704194249, 27.50000000000000355 ) ) ;
#8890=CARTESIAN_POINT ( 'NONE',  ( 29.61203839202725518, -15.40012917324033381, 41.62281023987508632 ) ) ;
#8891=CARTESIAN_POINT ( 'NONE',  ( -32.49058853941425440, -8.555876215535434426, 41.40177460044399993 ) ) ;
#8900=ORIENTED_EDGE ( 'NONE', *, *, #24351, .T. ) ;
#8901=CARTESIAN_POINT ( 'NONE',  ( 33.26833594138172145, 9.291422874672347731, 40.45861409864419045 ) ) ;
#8905=CARTESIAN_POINT ( 'NONE',  ( -27.03943647958861263, -26.20092231554396278, 34.80090346875804386 ) ) ;
#8926=CARTESIAN_POINT ( 'NONE',  ( 36.00000000000000000, -1.546978760965586295E-11, 34.75735931288068059 ) ) ;
#8927=CARTESIAN_POINT ( 'NONE',  ( 23.11524226670867321, -11.10088790631998634, 49.35779847069012050 ) ) ;
#8935=CARTESIAN_POINT ( 'NONE',  ( -3.431238874299064712, -42.34547772617858641, 28.85304416643127823 ) ) ;
#8961=CARTESIAN_POINT ( 'NONE',  ( 35.21442488810127713, -18.31310691302397231, 31.23994917172689156 ) ) ;
#8969=CARTESIAN_POINT ( 'NONE',  ( -18.17090117368252322, -32.80884700149822208, 37.50000000002933120 ) ) ;
#8977=EDGE_CURVE ( 'NONE', #3499, #3241, #9967, .T. ) ;
#8983=CYLINDRICAL_SURFACE ( 'NONE', #14779, 1.999999999999998224 ) ;
#8990=AXIS2_PLACEMENT_3D ( 'NONE', #3626, #29208, #1129 ) ;
#9028=CARTESIAN_POINT ( 'NONE',  ( 34.13832859401787800, -12.80067323710190053, 27.50000000000001776 ) ) ;
#9033=EDGE_CURVE ( 'NONE', #17339, #12561, #16883, .T. ) ;
#9048=FACE_BOUND ( 'NONE', #10031, .T. ) ;
#9052=CARTESIAN_POINT ( 'NONE',  ( -23.59263552078000359, 12.85968412197262545, 48.13036513616685141 ) ) ;
#9066=DIRECTION ( 'NONE',  ( -0.000000000000000000, -0.000000000000000000, -1.000000000000000000 ) ) ;
#9067=CARTESIAN_POINT ( 'NONE',  ( 35.89043209166288051, 3.548455793333529673, 34.73498294778850948 ) ) ;
#9082=CARTESIAN_POINT ( 'NONE',  ( 2.498618104684224850, -39.50000000000000000, 27.50000000000000711 ) ) ;
#9103=CARTESIAN_POINT ( 'NONE',  ( 12.79109178508979916, -40.15612306122757502, 29.04694596669003914 ) ) ;
#9114=CARTESIAN_POINT ( 'NONE',  ( 30.50257113119999275, -15.54031451041691803, 40.76699977199266556 ) ) ;
#9117=CARTESIAN_POINT ( 'NONE',  ( 23.59223810913926656, 12.86535672232149530, 43.88527982313174647 ) ) ;
#9136=CARTESIAN_POINT ( 'NONE',  ( 29.61203839202723032, 15.40012917324034092, -16.55003854064094426 ) ) ;
#9151=CARTESIAN_POINT ( 'NONE',  ( -33.32515425934906972, 22.24716177112028248, 34.67326153719451298 ) ) ;
#9212=CARTESIAN_POINT ( 'NONE',  ( -15.45157863257330533, 35.69925327167838702, 27.50000000000000711 ) ) ;
#9227=CARTESIAN_POINT ( 'NONE',  ( 35.56916886408897938, 6.214436617257074857, 27.50000000000000355 ) ) ;
#9230=B_SPLINE_CURVE_WITH_KNOTS ( 'NONE', 3,
 ( #10769, #22305, #8279, #948, #5634, #20281, #17638, #15130, #27308, #5475, #14976, #15434, #5938, #22455 ),
 .UNSPECIFIED., .F., .F.,
 ( 4, 2, 2, 2, 2, 2, 4 ),
 ( 2.111077618454142872E-07, 0.0004668847438969844690, 0.0009335583800321235227, 0.001400232016167262577, 0.001866905652302401630, 0.002800252924572683641, 0.003733600196842966085 ),
 .UNSPECIFIED. ) ;
#9234=DIRECTION ( 'NONE',  ( -0.000000000000000000, -0.000000000000000000, 1.000000000000000000 ) ) ;
#9253=CARTESIAN_POINT ( 'NONE',  ( 33.47974733229618494, -16.94066219419696750, 37.49999999993178079 ) ) ;
#9255=EDGE_LOOP ( 'NONE', ( #17915, #25671, #16416, #8067 ) ) ;
#9262=CARTESIAN_POINT ( 'NONE',  ( -31.79204601741444236, -14.90874471747207686, 35.64345580000767200 ) ) ;
#9264=EDGE_LOOP ( 'NONE', ( #1708, #12108, #30352, #16185 ) ) ;
#9272=CARTESIAN_POINT ( 'NONE',  ( -32.60829997825918980, -13.18983524832147936, 39.84356070656660620 ) ) ;
#9281=CARTESIAN_POINT ( 'NONE',  ( -4.163336342344337027E-14, 1.387778780781445676E-14, 34.49999999999999289 ) ) ;
#9299=CARTESIAN_POINT ( 'NONE',  ( -14.12911150912318803, 34.74147843573596361, 37.49999999997172040 ) ) ;
#9318=ORIENTED_EDGE ( 'NONE', *, *, #4812, .T. ) ;
#9322=AXIS2_PLACEMENT_3D ( 'NONE', #15729, #15899, #22593 ) ;
#9331=CARTESIAN_POINT ( 'NONE',  ( -4.163336342344337027E-14, 1.387778780781445676E-14, 62.49999999999999289 ) ) ;
#9356=CARTESIAN_POINT ( 'NONE',  ( 9.494436928264741837, -38.10466040143803212, 34.50000000000000000 ) ) ;
#9368=CARTESIAN_POINT ( 'NONE',  ( -35.89597485276235034, 3.063380141105419341, 27.49999999999999645 ) ) ;
#9387=CARTESIAN_POINT ( 'NONE',  ( 21.64339062281885973, -31.56738424159307499, 27.50000000000000711 ) ) ;
#9393=CARTESIAN_POINT ( 'NONE',  ( -31.57687401261850013, 15.10620312102103568, 39.99603010801635605 ) ) ;
#9416=CARTESIAN_POINT ( 'NONE',  ( 37.42187249122466142, 2.505710565345217855, 37.50000000001962519 ) ) ;
#9426=AXIS2_PLACEMENT_3D ( 'NONE', #4911, #2421, #5375 ) ;
#9446=CARTESIAN_POINT ( 'NONE',  ( -23.07950435457408034, -11.39185397358521001, 49.26234194702450964 ) ) ;
#9449=CARTESIAN_POINT ( 'NONE',  ( 33.56327786402390245, -10.34181101807379477, 35.63689980405263924 ) ) ;
#9454=DIRECTION ( 'NONE',  ( -0.000000000000000000, -0.000000000000000000, -1.000000000000000000 ) ) ;
#9465=CARTESIAN_POINT ( 'NONE',  ( -17.50822840077841747, 37.98520514636454948, 34.52714558546959012 ) ) ;
#9483=VERTEX_POINT ( 'NONE', #7961 ) ;
#9486=CARTESIAN_POINT ( 'NONE',  ( 0.000000000000000000, 0.000000000000000000, 0.000000000000000000 ) ) ;
#9488=CARTESIAN_POINT ( 'NONE',  ( -27.03074382657074537, -6.449748410230988327, -16.55003854064094426 ) ) ;
#9494=DIRECTION ( 'NONE',  ( -1.000000000000000000, 0.000000000000000000, 0.000000000000000000 ) ) ;
#9530=EDGE_CURVE ( 'NONE', #10675, #19313, #28546, .T. ) ;
#9532=CARTESIAN_POINT ( 'NONE',  ( 15.46896137236496216, 35.67159706264204999, 27.50000000000000711 ) ) ;
#9557=CARTESIAN_POINT ( 'NONE',  ( 35.66659450230903161, 17.24746242023032394, 34.79915034189033918 ) ) ;
#9570=ORIENTED_EDGE ( 'NONE', *, *, #3310, .T. ) ;
#9586=ADVANCED_FACE ( 'NONE', ( #27753 ), #25414, .F. ) ;
#9596=B_SPLINE_CURVE_WITH_KNOTS ( 'NONE', 3,
 ( #2410, #7403, #21727, #11936, #9727, #12081 ),
 .UNSPECIFIED., .F., .F.,
 ( 4, 2, 4 ),
 ( 2.108697328626194806E-07, 0.0003800081648695531069, 0.0007598054600062436074 ),
 .UNSPECIFIED. ) ;
#9601=LINE ( 'NONE', #20970, #29095 ) ;
#9603=CARTESIAN_POINT ( 'NONE',  ( -24.44496207165490276, 7.595930209050158588, 49.40206402021040333 ) ) ;
#9610=ORIENTED_EDGE ( 'NONE', *, *, #6527, .T. ) ;
#9615=CARTESIAN_POINT ( 'NONE',  ( -21.33648105846517495, 35.69619395329613099, 29.46852146853187193 ) ) ;
#9619=CARTESIAN_POINT ( 'NONE',  ( 33.21383100183306425, 9.208170138131603011, 36.29077426434711384 ) ) ;
#9623=CARTESIAN_POINT ( 'NONE',  ( 33.56327786402390245, -10.34181101807379655, -16.55003854064094426 ) ) ;
#9643=CARTESIAN_POINT ( 'NONE',  ( -30.33183837007556249, 13.53414739637282516, -16.55003854064094426 ) ) ;
#9661=FACE_OUTER_BOUND ( 'NONE', #6682, .T. ) ;
#9676=CARTESIAN_POINT ( 'NONE',  ( -33.53465676216265479, -14.39878183770549214, 34.49999999999997868 ) ) ;
#9685=CARTESIAN_POINT ( 'NONE',  ( 34.30746359002519341, 12.22650445617505355, 27.50000000000000711 ) ) ;
#9704=ORIENTED_EDGE ( 'NONE', *, *, #17818, .T. ) ;
#9705=CARTESIAN_POINT ( 'NONE',  ( 27.20641111072948348, 30.48549905497583978, 34.52784944976806258 ) ) ;
#9715=ORIENTED_EDGE ( 'NONE', *, *, #7117, .T. ) ;
#9719=ORIENTED_EDGE ( 'NONE', *, *, #19268, .T. ) ;
#9727=CARTESIAN_POINT ( 'NONE',  ( -23.07950435457408034, -11.39185397358521001, 45.01970125990521865 ) ) ;
#9730=EDGE_LOOP ( 'NONE', ( #26321, #1823, #10106, #23870 ) ) ;
#9751=CIRCLE ( 'NONE', #24184, 19.49999999999996447 ) ;
#9759=CARTESIAN_POINT ( 'NONE',  ( -38.60694528318246199, 6.056885966054946557, 35.03813756351178199 ) ) ;
#9763=EDGE_CURVE ( 'NONE', #13217, #28109, #27820, .T. ) ;
#9808=CARTESIAN_POINT ( 'NONE',  ( 38.85099238961694823, 3.925783015303134338, 32.18467226953571725 ) ) ;
#9826=CARTESIAN_POINT ( 'NONE',  ( 27.03074382657074537, 6.449748410230991880, -16.55003854064094426 ) ) ;
#9853=CARTESIAN_POINT ( 'NONE',  ( -4.272706734768118686, -37.25579118954082247, 37.50000000000000000 ) ) ;
#9868=CARTESIAN_POINT ( 'NONE',  ( 38.96687411310632854, 1.873333295377571650, 35.07604622541821726 ) ) ;
#9881=CARTESIAN_POINT ( 'NONE',  ( 0.000000000000000000, 39.50000000000000000, 34.49999999999999289 ) ) ;
#9899=CARTESIAN_POINT ( 'NONE',  ( -37.50000000000005684, 9.285362311011880811E-15, 37.50000000000000000 ) ) ;
#9919=CARTESIAN_POINT ( 'NONE',  ( -22.70739019994807251, -29.86753719045417910, 37.49999999998765077 ) ) ;
#9921=DIRECTION ( 'NONE',  ( -0.000000000000000000, -0.000000000000000000, 1.000000000000000000 ) ) ;
#9957=CARTESIAN_POINT ( 'NONE',  ( -26.58597676761596063, 6.321098805557480382, 47.67294373134352270 ) ) ;
#9963=EDGE_CURVE ( 'NONE', #28104, #19006, #6207, .T. ) ;
#9967=B_SPLINE_CURVE_WITH_KNOTS ( 'NONE', 3,
 ( #26746, #5068, #2251, #30798, #9446, #16603 ),
 .UNSPECIFIED., .F., .F.,
 ( 4, 2, 4 ),
 ( 2.108697328626194806E-07, 0.0003800081648695531611, 0.0007598054600062437158 ),
 .UNSPECIFIED. ) ;
#9975=CARTESIAN_POINT ( 'NONE',  ( -24.57665676473017413, -33.00632471879952590, 29.73950062350330725 ) ) ;
#10008=CARTESIAN_POINT ( 'NONE',  ( 33.42925964089140933, 11.06161099612213405, 39.78814634291935448 ) ) ;
#10012=CARTESIAN_POINT ( 'NONE',  ( 33.47438960496221227, 10.94461781313380477, 39.78205384324066074 ) ) ;
#10015=B_SPLINE_CURVE_WITH_KNOTS ( 'NONE', 3,
 ( #30135, #18290, #10648, #11262 ),
 .UNSPECIFIED., .F., .F.,
 ( 4, 4 ),
 ( 3.022186913359086288E-07, 0.007932103869840194041 ),
 .UNSPECIFIED. ) ;
#10025=CARTESIAN_POINT ( 'NONE',  ( 28.00167021653412291, 24.95069493026310070, 37.49999999999567990 ) ) ;
#10027=DIRECTION ( 'NONE',  ( 1.000000000000000000, 0.000000000000000000, 0.000000000000000000 ) ) ;
#10031=EDGE_LOOP ( 'NONE', ( #25902, #22592, #17073, #23545, #5974, #6725, #8022, #12333, #8900 ) ) ;
#10040=CARTESIAN_POINT ( 'NONE',  ( -29.55190575096636607, 22.57725177722917920, 34.50000000000000711 ) ) ;
#10056=VERTEX_POINT ( 'NONE', #20329 ) ;
#10062=ORIENTED_EDGE ( 'NONE', *, *, #13390, .T. ) ;
#10067=CARTESIAN_POINT ( 'NONE',  ( -24.03448224033878944, -8.660042335149837456, 45.23564988763774863 ) ) ;
#10071=CARTESIAN_POINT ( 'NONE',  ( -29.86178407246424626, -27.47635996432160255, 34.56532846876351073 ) ) ;
#10088=ORIENTED_EDGE ( 'NONE', *, *, #15880, .T. ) ;
#10092=FACE_BOUND ( 'NONE', #28857, .T. ) ;
#10106=ORIENTED_EDGE ( 'NONE', *, *, #15231, .T. ) ;
#10107=B_SPLINE_CURVE_WITH_KNOTS ( 'NONE', 3,
 ( #11249, #30429, #1734, #13898 ),
 .UNSPECIFIED., .F., .F.,
 ( 4, 4 ),
 ( 3.022186913382060468E-07, 0.007932103869840216592 ),
 .UNSPECIFIED. ) ;
#10109=CARTESIAN_POINT ( 'NONE',  ( 35.53662292511247500, 17.55688491361479819, 31.31080097343302171 ) ) ;
#10113=CARTESIAN_POINT ( 'NONE',  ( -25.05233252773468422, -32.57872576663409347, 29.78309721723623582 ) ) ;
#10115=FACE_OUTER_BOUND ( 'NONE', #25680, .T. ) ;
#10120=CARTESIAN_POINT ( 'NONE',  ( 28.69771818040356237, -23.84998595875660499, 34.50000000000000711 ) ) ;
#10125=EDGE_CURVE ( 'NONE', #4914, #4107, #4702, .T. ) ;
#10145=CARTESIAN_POINT ( 'NONE',  ( 25.07950435457407323, 11.50806656539753270, -16.55003854064094426 ) ) ;
#10146=CARTESIAN_POINT ( 'NONE',  ( -24.44496207165490276, 7.595930209050158588, 45.15942333309111945 ) ) ;
#10147=ORIENTED_EDGE ( 'NONE', *, *, #10940, .F. ) ;
#10150=CARTESIAN_POINT ( 'NONE',  ( -27.03074382657074537, -6.449748410230988327, 42.96778633356042576 ) ) ;
#10153=CARTESIAN_POINT ( 'NONE',  ( -2.338573377552018773, 39.50000000000000711, 34.80090346875804386 ) ) ;
#10155=CARTESIAN_POINT ( 'NONE',  ( 32.14095006730908466, 14.40137518142634043, 39.78046893946842744 ) ) ;
#10171=CARTESIAN_POINT ( 'NONE',  ( 12.18627938514990383, 35.48392282099285211, 37.50000000002605560 ) ) ;
#10188=CARTESIAN_POINT ( 'NONE',  ( 26.31094384852241319, -8.315730187098496984, -16.55003854064094426 ) ) ;
#10189=CARTESIAN_POINT ( 'NONE',  ( -34.70577939417217550, -10.49309206032214270, 34.49999999999999289 ) ) ;
#10195=DIRECTION ( 'NONE',  ( 1.000000000000000000, 0.000000000000000000, 0.000000000000000000 ) ) ;
#10216=B_SPLINE_CURVE_WITH_KNOTS ( 'NONE', 3,
 ( #22752, #4341, #18089, #17943, #13867, #25102, #1558, #8435, #23369, #30242, #25419, #10756, #3745, #13570 ),
 .UNSPECIFIED., .F., .F.,
 ( 4, 2, 2, 2, 2, 2, 4 ),
 ( 2.108697328626194806E-07, 0.0004867403590529696938, 0.0009732698483730767812, 0.001459799337693183652, 0.001946328827013290956, 0.002919387805653491253, 0.003892446784293692418 ),
 .UNSPECIFIED. ) ;
#10220=CARTESIAN_POINT ( 'NONE',  ( -39.02702558981775383, 2.049152216486670230, 32.23957365480787729 ) ) ;
#10228=CARTESIAN_POINT ( 'NONE',  ( 30.03792366816883330, 15.52577997660843145, 36.94438844912271946 ) ) ;
#10229=ADVANCED_FACE ( 'NONE', ( #21144 ), #13700, .F. ) ;
#10242=FACE_BOUND ( 'NONE', #19083, .T. ) ;
#10259=CARTESIAN_POINT ( 'NONE',  ( 37.60443094512424977, -11.34029379291156836, 31.81961544519251106 ) ) ;
#10263=VECTOR ( 'NONE', #18682, 1000.000000000000000 ) ;
#10264=CARTESIAN_POINT ( 'NONE',  ( -39.07074351764322984, -0.08311056096719925124, 32.25448628877133217 ) ) ;
#10265=CARTESIAN_POINT ( 'NONE',  ( 0.000000000000000000, 42.50000000000000000, 32.26246401786215046 ) ) ;
#10301=ADVANCED_FACE ( 'NONE', ( #13552, #16180, #25855 ), #5311, .F. ) ;
#10310=CARTESIAN_POINT ( 'NONE',  ( 33.56327786402390245, 10.34181101807379299, 39.87954049117193023 ) ) ;
#10313=CARTESIAN_POINT ( 'NONE',  ( -26.12638453225887503, -6.310846377660610962, 48.12226976367811204 ) ) ;
#10332=AXIS2_PLACEMENT_3D ( 'NONE', #1269, #11398, #27319 ) ;
#10345=AXIS2_PLACEMENT_3D ( 'NONE', #26932, #3363, #1031 ) ;
#10347=CARTESIAN_POINT ( 'NONE',  ( -32.99407928578143867, 15.80558523611060018, 34.49999999999998579 ) ) ;
#10356=FACE_OUTER_BOUND ( 'NONE', #24128, .T. ) ;
#10374=CARTESIAN_POINT ( 'NONE',  ( 2.161275096740449708, -37.44220553068277724, 37.50000000000981260 ) ) ;
#10386=CARTESIAN_POINT ( 'NONE',  ( -33.10232066993145139, -22.48641252920058164, 34.66925410237854521 ) ) ;
#10403=ORIENTED_EDGE ( 'NONE', *, *, #18176, .F. ) ;
#10434=CARTESIAN_POINT ( 'NONE',  ( -5.145204076156935535, 42.13436674946195382, 28.87129565651644825 ) ) ;
#10440=CARTESIAN_POINT ( 'NONE',  ( 28.98606489759778881, -23.42647331253649412, 34.50000000000000000 ) ) ;
#10456=EDGE_LOOP ( 'NONE', ( #28585, #11923, #20364, #22868, #28157, #20973, #27645 ) ) ;
#10467=CARTESIAN_POINT ( 'NONE',  ( 13.79614740859419797, 36.49939583300671586, 34.49999999999999289 ) ) ;
#10468=CARTESIAN_POINT ( 'NONE',  ( -27.03943647958860552, 26.20092231554396633, 27.50000000000001066 ) ) ;
#10470=CARTESIAN_POINT ( 'NONE',  ( 33.55235357430897380, 10.58403138555777900, 39.81808279656205229 ) ) ;
#10473=AXIS2_PLACEMENT_3D ( 'NONE', #19502, #2347, #29013 ) ;
#10480=CARTESIAN_POINT ( 'NONE',  ( -24.18511243334008043, -13.30669973338235401, 47.39588261142744585 ) ) ;
#10486=CARTESIAN_POINT ( 'NONE',  ( 4.216636297896264374, 37.26217892624189432, 37.50000000000000000 ) ) ;
#10489=CARTESIAN_POINT ( 'NONE',  ( 25.88640477275122365, 6.345529225273955021, 44.10491087709814906 ) ) ;
#10500=CARTESIAN_POINT ( 'NONE',  ( -34.45952885238020258, 11.47311510027356007, 34.50000000000000711 ) ) ;
#10508=( NAMED_UNIT ( * ) PLANE_ANGLE_UNIT ( ) SI_UNIT ( $, .RADIAN. ) );
#10516=CARTESIAN_POINT ( 'NONE',  ( 33.55224573311710401, -10.10291939066352640, 35.71721447083890411 ) ) ;
#10521=EDGE_CURVE ( 'NONE', #23899, #30628, #3534, .T. ) ;
#10522=CARTESIAN_POINT ( 'NONE',  ( 5.068365686548764515, -37.22901435740217124, 37.49999999996078515 ) ) ;
#10534=CARTESIAN_POINT ( 'NONE',  ( -36.28305795128277111, -9.498090346893212299, 37.50000000001156053 ) ) ;
#10535=ORIENTED_EDGE ( 'NONE', *, *, #10890, .T. ) ;
#10564=( LENGTH_UNIT ( ) NAMED_UNIT ( * ) SI_UNIT ( .MILLI., .METRE. ) );
#10568=EDGE_LOOP ( 'NONE', ( #22095, #13062 ) ) ;
#10581=CARTESIAN_POINT ( 'NONE',  ( 28.21921180493569281, -29.36589712660545359, 30.11501300312919938 ) ) ;
#10585=CARTESIAN_POINT ( 'NONE',  ( -38.72977682550716594, 5.035713241503631643, 32.14724780218217859 ) ) ;
#10595=ORIENTED_EDGE ( 'NONE', *, *, #22971, .F. ) ;
#10626=CARTESIAN_POINT ( 'NONE',  ( 27.03074382657074537, 6.449748410230989215, 47.21042702067963148 ) ) ;
#10639=VECTOR ( 'NONE', #18271, 1000.000000000000000 ) ;
#10640=CARTESIAN_POINT ( 'NONE',  ( 17.09492967699473809, 33.38213141764304481, 37.50000000000831335 ) ) ;
#10648=CARTESIAN_POINT ( 'NONE',  ( -28.78283879316666471, -7.125616703334841873, 41.10667063058298965 ) ) ;
#10671=CARTESIAN_POINT ( 'NONE',  ( -31.46108752401732289, 15.19043599309334702, 35.82118098715100984 ) ) ;
#10675=VERTEX_POINT ( 'NONE', #22999 ) ;
#10676=CARTESIAN_POINT ( 'NONE',  ( 29.61203839202723032, 15.40012917324034092, 37.38016955275583797 ) ) ;
#10707=EDGE_LOOP ( 'NONE', ( #17588, #22895, #25552, #13013 ) ) ;
#10744=CARTESIAN_POINT ( 'NONE',  ( 28.55068628633582151, 24.19494186940699620, 27.50000000000000355 ) ) ;
#10745=ORIENTED_EDGE ( 'NONE', *, *, #30325, .F. ) ;
#10756=CARTESIAN_POINT ( 'NONE',  ( 23.94376008874366235, 13.17067969463889732, 47.67294373119254658 ) ) ;
#10769=CARTESIAN_POINT ( 'NONE',  ( 32.19782014694308003, -14.25394737442115201, 35.54550565580006349 ) ) ;
#10776=CARTESIAN_POINT ( 'NONE',  ( -32.31576317091163730, -17.59561277345963148, 27.50000000000000355 ) ) ;
#10810=CARTESIAN_POINT ( 'NONE',  ( 13.24704986988986199, -36.75107818987552832, 27.50000000000000355 ) ) ;
#10820=( LENGTH_UNIT ( ) NAMED_UNIT ( * ) SI_UNIT ( .MILLI., .METRE. ) );
#10824=B_SPLINE_CURVE_WITH_KNOTS ( 'NONE', 3,
 ( #5943, #12968, #22459, #20132, #1575, #13277, #29814, #8901, #8596, #8456, #15923, #29649, #8285, #13587 ),
 .UNSPECIFIED., .F., .F.,
 ( 4, 2, 2, 2, 2, 2, 4 ),
 ( 0.0007411796533686801358, 0.001115232222424167698, 0.001489284791479655260, 0.001863337360535142605, 0.002237389929590630384, 0.002985495067701605075, 0.003733600205812580199 ),
 .UNSPECIFIED. ) ;
#10846=ORIENTED_EDGE ( 'NONE', *, *, #2346, .F. ) ;
#10847=CARTESIAN_POINT ( 'NONE',  ( 24.44496207165490276, 7.595930209050162141, -16.55003854064094426 ) ) ;
#10848=CARTESIAN_POINT ( 'NONE',  ( -6.513023399507313904, -41.93085199890154513, 28.88895809215988919 ) ) ;
#10855=CARTESIAN_POINT ( 'NONE',  ( 23.44138668973443629, 12.68271180600416237, 44.10533075972621475 ) ) ;
#10862=CARTESIAN_POINT ( 'NONE',  ( -4.163336342344337027E-14, 1.387778780781445676E-14, 62.49999999999999289 ) ) ;
#10866=CARTESIAN_POINT ( 'NONE',  ( 34.70577939417261604, -10.49309206032036634, 34.49999999999999289 ) ) ;
#10874=VERTEX_POINT ( 'NONE', #12820 ) ;
#10875=CIRCLE ( 'NONE', #21812, 22.49999999999996447 ) ;
#10882=CARTESIAN_POINT ( 'NONE',  ( -31.89119714134806927, -14.79609055705960863, 35.60128781023438194 ) ) ;
#10886=CARTESIAN_POINT ( 'NONE',  ( -15.96900124075088456, 38.78095776257472949, 29.17368192679814243 ) ) ;
#10890=EDGE_CURVE ( 'NONE', #20928, #3711, #16580, .T. ) ;
#10891=FACE_OUTER_BOUND ( 'NONE', #18268, .T. ) ;
#10912=CARTESIAN_POINT ( 'NONE',  ( 28.55068628633582151, 24.19494186940699620, 34.80090346875809360 ) ) ;
#10917=B_SPLINE_CURVE_WITH_KNOTS ( 'NONE', 3,
 ( #15583, #18088, #6680, #13261 ),
 .UNSPECIFIED., .F., .F.,
 ( 4, 4 ),
 ( 3.022186913382060468E-07, 0.007932103869840195776 ),
 .UNSPECIFIED. ) ;
#10921=DIRECTION ( 'NONE',  ( 1.000000000000000000, 0.000000000000000000, 0.000000000000000000 ) ) ;
#10923=CARTESIAN_POINT ( 'NONE',  ( -32.19782014694307293, -14.25394737442115733, 35.54550565580014876 ) ) ;
#10939=EDGE_CURVE ( 'NONE', #11554, #18416, #6923, .T. ) ;
#10940=EDGE_CURVE ( 'NONE', #6144, #11315, #22622, .T. ) ;
#10953=VERTEX_POINT ( 'NONE', #3765 ) ;
#10966=CARTESIAN_POINT ( 'NONE',  ( -33.19297012087366028, -9.154531925606914200, 36.32560960716998011 ) ) ;
#10985=CARTESIAN_POINT ( 'NONE',  ( -27.03074382657074537, -6.449748410230988327, -16.55003854064094426 ) ) ;
#10990=DIRECTION ( 'NONE',  ( -0.000000000000000000, -0.000000000000000000, 1.000000000000000000 ) ) ;
#10995=CARTESIAN_POINT ( 'NONE',  ( 36.61818605946716332, -14.68367171281316175, 31.56304765520175692 ) ) ;
#11007=CARTESIAN_POINT ( 'NONE',  ( 31.46108752401734066, -15.19043599309334169, 40.06382167427020136 ) ) ;
#11035=CARTESIAN_POINT ( 'NONE',  ( -32.19782014694307293, -14.25394737442115733, 35.54550565580014876 ) ) ;
#11039=ORIENTED_EDGE ( 'NONE', *, *, #13448, .T. ) ;
#11041=ORIENTED_EDGE ( 'NONE', *, *, #19663, .F. ) ;
#11047=CARTESIAN_POINT ( 'NONE',  ( 29.04733024409324571, -28.39068243925979473, 30.21700144173808411 ) ) ;
#11056=CARTESIAN_POINT ( 'NONE',  ( 17.94248964168179583, 34.33858135081683827, 27.50000000000000355 ) ) ;
#11070=CARTESIAN_POINT ( 'NONE',  ( 31.56327786402390245, -10.34181101807379655, -16.55003854064094426 ) ) ;
#11086=CARTESIAN_POINT ( 'NONE',  ( -21.86019681245147694, -31.48592878035298170, 34.80090346875804386 ) ) ;
#11087=FACE_OUTER_BOUND ( 'NONE', #5116, .T. ) ;
#11089=ADVANCED_FACE ( 'NONE', ( #9661 ), #18876, .F. ) ;
#11116=EDGE_CURVE ( 'NONE', #20027, #1048, #1343, .T. ) ;
#11117=VERTEX_POINT ( 'NONE', #7502 ) ;
#11129=CARTESIAN_POINT ( 'NONE',  ( -32.19782014694307293, 14.25394737442115733, 39.78814634291943975 ) ) ;
#11145=CARTESIAN_POINT ( 'NONE',  ( 33.55102796320213798, -21.82697637830245085, 30.90080749576968699 ) ) ;
#11177=AXIS2_PLACEMENT_3D ( 'NONE', #9331, #7462, #14011 ) ;
#11180=B_SPLINE_CURVE_WITH_KNOTS ( 'NONE', 3,
 ( #4365, #2024, #11551, #21041, #25891, #9356, #30563, #23681, #6856, #28390, #7015, #16524, #2326, #21353, #16983, #17139, #295, #29315, #749, #10120, #10440, #14957, #24468, #24149, #3113, #12633, #22122, #5136, #5609, #26983 ),
 .UNSPECIFIED., .F., .F.,
 ( 4, 2, 2, 2, 2, 2, 2, 2, 2, 2, 2, 2, 2, 2, 4 ),
 ( 0.000000000000000000, 0.006058912026177337706, 0.009088368039266010029, 0.01060309604581034446, 0.01211782405235468062, 0.01817673607853203394, 0.02120619209162071667, 0.02423564810470939940, 0.03029456013088676139, 0.03332401614397544759, 0.03483874415051978202, 0.03635347215706412338, 0.04241238418324148884, 0.04544184019633017851, 0.04847129620941885431 ),
 .UNSPECIFIED. ) ;
#11187=CARTESIAN_POINT ( 'NONE',  ( -6.091847012640411840, 42.00621603651080704, 28.88234630096432554 ) ) ;
#11197=CARTESIAN_POINT ( 'NONE',  ( 30.22537216192871057, -26.86607088810509936, 30.37637886334946558 ) ) ;
#11206=CARTESIAN_POINT ( 'NONE',  ( 27.03943647958860197, -26.20092231554396633, 27.50000000000001066 ) ) ;
#11215=CARTESIAN_POINT ( 'NONE',  ( -30.53339558441486190, 7.800891647352838909, 43.48653168448687012 ) ) ;
#11217=DIRECTION ( 'NONE',  ( -0.000000000000000000, -0.000000000000000000, 1.000000000000000000 ) ) ;
#11219=CARTESIAN_POINT ( 'NONE',  ( -33.42925964089141644, -11.06161099612212695, 39.78814634291941843 ) ) ;
#11231=CARTESIAN_POINT ( 'NONE',  ( -34.13832859401788511, 12.80067323710188276, 34.80090346875805807 ) ) ;
#11232=CARTESIAN_POINT ( 'NONE',  ( -27.03074382657074537, 6.449748410230984774, 42.96778633356043287 ) ) ;
#11249=CARTESIAN_POINT ( 'NONE',  ( 29.61203839202725518, -15.40012917324033381, 37.38016955275580244 ) ) ;
#11253=CYLINDRICAL_SURFACE ( 'NONE', #16195, 19.49999999999996447 ) ;
#11254=CARTESIAN_POINT ( 'NONE',  ( 27.03074382657074537, 6.449748410230989215, 47.21042702067963148 ) ) ;
#11256=AXIS2_PLACEMENT_3D ( 'NONE', #23480, #16936, #26454 ) ;
#11260=ADVANCED_FACE ( 'NONE', ( #15586 ), #20428, .F. ) ;
#11262=CARTESIAN_POINT ( 'NONE',  ( -27.03074382657074537, -6.449748410230988327, 42.96778633356042576 ) ) ;
#11282=CARTESIAN_POINT ( 'NONE',  ( -23.07950435457407679, -11.50806656539752737, -16.55003854064094426 ) ) ;
#11290=ORIENTED_EDGE ( 'NONE', *, *, #21603, .F. ) ;
#11293=CARTESIAN_POINT ( 'NONE',  ( 30.96729785525396395, -21.29736153647971619, 37.49999999991082689 ) ) ;
#11304=ADVANCED_FACE ( 'NONE', ( #16198 ), #13574, .F. ) ;
#11308=CARTESIAN_POINT ( 'NONE',  ( -30.74147208807243814, -15.49548351932574697, 40.57409041152976670 ) ) ;
#11310=AXIS2_PLACEMENT_3D ( 'NONE', #13996, #27738, #13851 ) ;
#11315=VERTEX_POINT ( 'NONE', #8890 ) ;
#11318=CARTESIAN_POINT ( 'NONE',  ( -4.163336342344337027E-14, 1.387778780781445676E-14, 62.49999999999999289 ) ) ;
#11334=CARTESIAN_POINT ( 'NONE',  ( 33.42925964089140933, 11.06161099612213405, -16.55003854064094426 ) ) ;
#11337=CARTESIAN_POINT ( 'NONE',  ( 0.000000000000000000, 39.50000000000000000, 37.50000000000000000 ) ) ;
#11347=VECTOR ( 'NONE', #170, 1000.000000000000000 ) ;
#11350=CARTESIAN_POINT ( 'NONE',  ( -14.09828636627701925, 39.65347080688651715, 29.09260480754099021 ) ) ;
#11353=ORIENTED_EDGE ( 'NONE', *, *, #26337, .T. ) ;
#11372=FACE_OUTER_BOUND ( 'NONE', #12158, .T. ) ;
#11378=AXIS2_PLACEMENT_3D ( 'NONE', #10145, #24169, #25803 ) ;
#11387=VERTEX_POINT ( 'NONE', #20714 ) ;
#11397=CARTESIAN_POINT ( 'NONE',  ( -32.31576317091163730, -17.59561277345963148, 34.80090346875804386 ) ) ;
#11398=DIRECTION ( 'NONE',  ( -0.000000000000000000, -0.000000000000000000, 1.000000000000000000 ) ) ;
#11415=CARTESIAN_POINT ( 'NONE',  ( -12.08674330573844813, 37.23003549701822834, 27.50000000000000355 ) ) ;
#11417=CARTESIAN_POINT ( 'NONE',  ( 23.21352257770656635, -10.78826658734920052, 49.40206402021031806 ) ) ;
#11437=ORIENTED_EDGE ( 'NONE', *, *, #3732, .T. ) ;
#11451=CARTESIAN_POINT ( 'NONE',  ( 24.35498655531922196, -28.61621432983365665, 37.50000000002946621 ) ) ;
#11475=DIRECTION ( 'NONE',  ( -0.000000000000000000, -0.000000000000000000, 1.000000000000000000 ) ) ;
#11501=CARTESIAN_POINT ( 'NONE',  ( -0.5346017343310117687, 42.60462856552967281, 28.83069491023030295 ) ) ;
#11515=CARTESIAN_POINT ( 'NONE',  ( 25.07174449839132180, -6.739288358966156522, 49.03857552305933609 ) ) ;
#11523=CARTESIAN_POINT ( 'NONE',  ( -29.61203839202723032, -15.40012917324033381, -16.55003854064094426 ) ) ;
#11533=ORIENTED_EDGE ( 'NONE', *, *, #23307, .T. ) ;
#11543=FACE_OUTER_BOUND ( 'NONE', #1986, .T. ) ;
#11551=CARTESIAN_POINT ( 'NONE',  ( 4.066382127562278015, -39.30923493945141445, 34.49999999999999289 ) ) ;
#11554=VERTEX_POINT ( 'NONE', #26963 ) ;
#11571=CARTESIAN_POINT ( 'NONE',  ( 26.86404174848737725, -26.32179565544504030, 27.50000000000000711 ) ) ;
#11580=ORIENTED_EDGE ( 'NONE', *, *, #587, .T. ) ;
#11588=ORIENTED_EDGE ( 'NONE', *, *, #807, .T. ) ;
#11593=CARTESIAN_POINT ( 'NONE',  ( 33.33631137181001236, -22.22424899003631182, 34.67383366597271532 ) ) ;
#11600=ORIENTED_EDGE ( 'NONE', *, *, #17933, .T. ) ;
#11615=CARTESIAN_POINT ( 'NONE',  ( 28.78283879316666471, 7.125616703334846314, 41.10667063058291149 ) ) ;
#11639=EDGE_CURVE ( 'NONE', #29565, #23323, #23194, .T. ) ;
#11641=CARTESIAN_POINT ( 'NONE',  ( -35.21927848278606632, 18.30290806334510023, 31.24093525326876275 ) ) ;
#11648=ORIENTED_EDGE ( 'NONE', *, *, #18891, .T. ) ;
#11689=CARTESIAN_POINT ( 'NONE',  ( -5.127072262013854242, -42.13114360820154047, 28.87158698979397897 ) ) ;
#11694=DIRECTION ( 'NONE',  ( 0.9329908884337534403, 0.3598999890241668664, 0.000000000000000000 ) ) ;
#11706=CARTESIAN_POINT ( 'NONE',  ( 0.000000000000000000, 39.50000000000000000, 27.50000000000000355 ) ) ;
#11720=CARTESIAN_POINT ( 'NONE',  ( 35.99942728066312725, 0.6588716437970913997, 27.50000000000001066 ) ) ;
#11744=CARTESIAN_POINT ( 'NONE',  ( 30.38390623893337761, 22.11697395215319162, 37.50000000001698197 ) ) ;
#11747=VECTOR ( 'NONE', #24969, 1000.000000000000000 ) ;
#11763=CARTESIAN_POINT ( 'NONE',  ( 29.61203839202722676, 15.40012917324034092, 41.62281023987512185 ) ) ;
#11774=CARTESIAN_POINT ( 'NONE',  ( 33.03549465208794800, -8.974030344605379739, 36.52487348530875266 ) ) ;
#11792=CARTESIAN_POINT ( 'NONE',  ( -25.91933551046517081, 31.76379658186127841, 29.86662960453368143 ) ) ;
#11834=CARTESIAN_POINT ( 'NONE',  ( -24.75800239156184190, 7.045788922043114688, 49.25937209215337020 ) ) ;
#11842=VECTOR ( 'NONE', #15357, 1000.000000000000000 ) ;
#11843=CARTESIAN_POINT ( 'NONE',  ( -4.163336342344337027E-14, 1.387778780781445676E-14, 37.50000000000000000 ) ) ;
#11846=CIRCLE ( 'NONE', #22800, 19.49999999999996447 ) ;
#11848=CARTESIAN_POINT ( 'NONE',  ( -10.15881039258890794, -41.03878892760899078, 28.96756984954204839 ) ) ;
#11861=DIRECTION ( 'NONE',  ( 1.000000000000000000, 0.000000000000000000, -0.000000000000000000 ) ) ;
#11863=FACE_OUTER_BOUND ( 'NONE', #18075, .T. ) ;
#11868=CARTESIAN_POINT ( 'NONE',  ( -4.346265761537661199, -39.21681178834676018, 27.50000000000000355 ) ) ;
#11874=CARTESIAN_POINT ( 'NONE',  ( -34.45740060152252227, -11.48158507098138692, 34.49999999999999289 ) ) ;
#11881=ORIENTED_EDGE ( 'NONE', *, *, #2938, .F. ) ;
#11887=CARTESIAN_POINT ( 'NONE',  ( 29.06267346339080504, -23.31480175602749938, 27.50000000000000355 ) ) ;
#11906=DIRECTION ( 'NONE',  ( 1.000000000000000000, 0.000000000000000000, 0.000000000000000000 ) ) ;
#11911=ORIENTED_EDGE ( 'NONE', *, *, #2312, .T. ) ;
#11914=CARTESIAN_POINT ( 'NONE',  ( 31.78338042482835846, 20.06055218721173006, 37.49999999987489474 ) ) ;
#11923=ORIENTED_EDGE ( 'NONE', *, *, #13186, .T. ) ;
#11936=CARTESIAN_POINT ( 'NONE',  ( -23.08991993893192785, -11.27014480227852644, 45.06404153503662258 ) ) ;
#11964=CARTESIAN_POINT ( 'NONE',  ( -30.95493403226913998, 21.31809426914557193, 37.49999999984183319 ) ) ;
#11993=CARTESIAN_POINT ( 'NONE',  ( -24.57973596967191554, 7.302173446879558938, 49.35895363830209703 ) ) ;
#11994=ORIENTED_EDGE ( 'NONE', *, *, #28805, .T. ) ;
#11995=CARTESIAN_POINT ( 'NONE',  ( 24.14264434021282213, -13.29031772318284865, 43.19835251277588384 ) ) ;
#11997=ORIENTED_EDGE ( 'NONE', *, *, #26946, .T. ) ;
#12009=CARTESIAN_POINT ( 'NONE',  ( -24.35970437652574105, -13.37404834226503247, -16.55003854064094426 ) ) ;
#12019=CARTESIAN_POINT ( 'NONE',  ( -33.87117184736123221, -13.39279440468763660, 27.50000000000000711 ) ) ;
#12023=CARTESIAN_POINT ( 'NONE',  ( -4.082808312865499722, -39.26097399651455788, 34.49999999999998579 ) ) ;
#12034=CARTESIAN_POINT ( 'NONE',  ( 35.16664802458688399, -8.537212109034927110, 27.50000000000000355 ) ) ;
#12035=EDGE_CURVE ( 'NONE', #17814, #4181, #5757, .T. ) ;
#12041=CARTESIAN_POINT ( 'NONE',  ( 33.56327786402390245, -10.34181101807379477, 39.87954049117192312 ) ) ;
#12044=AXIS2_PLACEMENT_3D ( 'NONE', #21816, #28992, #5285 ) ;
#12060=CARTESIAN_POINT ( 'NONE',  ( 36.26666421214746094, 15.68564761223754900, 31.47842155818181809 ) ) ;
#12081=CARTESIAN_POINT ( 'NONE',  ( -23.07950435457407679, -11.50806656539752737, 44.96784366550136980 ) ) ;
#12108=ORIENTED_EDGE ( 'NONE', *, *, #20624, .T. ) ;
#12113=CARTESIAN_POINT ( 'NONE',  ( -36.66434526847238828, 7.899044488850192280, 37.50000000002572875 ) ) ;
#12131=LINE ( 'NONE', #11523, #1636 ) ;
#12134=AXIS2_PLACEMENT_3D ( 'NONE', #30715, #21665, #11861 ) ;
#12145=CARTESIAN_POINT ( 'NONE',  ( -24.50429677314016175, 7.442113211156454078, 49.39104550111589020 ) ) ;
#12152=CARTESIAN_POINT ( 'NONE',  ( 36.45295081748523103, 15.16267811623469974, 31.52271926598579199 ) ) ;
#12156=CARTESIAN_POINT ( 'NONE',  ( -24.02386986937632685, 13.21681873352653014, 47.58048285248938214 ) ) ;
#12158=EDGE_LOOP ( 'NONE', ( #6099, #20443, #12932, #16322, #29734, #6788, #26475 ) ) ;
#12171=AXIS2_PLACEMENT_3D ( 'NONE', #9643, #19154, #7302 ) ;
#12175=CARTESIAN_POINT ( 'NONE',  ( -33.18278998769607568, -15.34828001744181059, 34.50000000000000000 ) ) ;
#12195=DIRECTION ( 'NONE',  ( -0.3598999890241700306, -0.9329908884337522190, 0.000000000000000000 ) ) ;
#12203=CARTESIAN_POINT ( 'NONE',  ( 35.55342103166282897, 11.99406784226782108, 37.49999999999405276 ) ) ;
#12209=CARTESIAN_POINT ( 'NONE',  ( -24.18511243334008043, -13.30669973338235401, 43.15324192430815486 ) ) ;
#12220=CARTESIAN_POINT ( 'NONE',  ( -23.07950435457394889, 11.39182330144667432, 49.26235563386612171 ) ) ;
#12246=EDGE_CURVE ( 'NONE', #438, #2953, #6399, .T. ) ;
#12255=EDGE_LOOP ( 'NONE', ( #14802, #25650 ) ) ;
#12260=CARTESIAN_POINT ( 'NONE',  ( -36.59094164303683527, -8.232679042141276327, 37.49999999998843947 ) ) ;
#12269=FACE_OUTER_BOUND ( 'NONE', #12601, .T. ) ;
#12282=EDGE_CURVE ( 'NONE', #22753, #27284, #30099, .T. ) ;
#12288=CARTESIAN_POINT ( 'NONE',  ( -4.163336342344337027E-14, 1.387778780781445676E-14, 35.37867965644034740 ) ) ;
#12301=ORIENTED_EDGE ( 'NONE', *, *, #10125, .T. ) ;
#12311=CARTESIAN_POINT ( 'NONE',  ( -34.55261918705283364, 19.75278628345992260, 31.10207979175319437 ) ) ;
#12330=B_SPLINE_CURVE_WITH_KNOTS ( 'NONE', 3,
 ( #1452, #3312, #5970, #27030, #20000, #8618, #1287, #25300, #12841, #10966, #17661, #29985, #27642, #15467 ),
 .UNSPECIFIED., .F., .F.,
 ( 4, 2, 2, 2, 2, 2, 4 ),
 ( 2.111164903073641426E-07, 0.0004668847526555941377, 0.0009335583888208808965, 0.001400232024986167601, 0.001866905661151454414, 0.002800252933482019584, 0.003733600205812584970 ),
 .UNSPECIFIED. ) ;
#12333=ORIENTED_EDGE ( 'NONE', *, *, #3267, .T. ) ;
#12336=CARTESIAN_POINT ( 'NONE',  ( -26.87942847751985909, -26.27672867733070206, 34.50000000000000711 ) ) ;
#12349=DIRECTION ( 'NONE',  ( -0.000000000000000000, -0.000000000000000000, 1.000000000000000000 ) ) ;
#12369=CARTESIAN_POINT ( 'NONE',  ( 39.00438428794741696, -0.1180012993332143073, 32.23357027876486569 ) ) ;
#12385=CARTESIAN_POINT ( 'NONE',  ( -33.18055756306304716, 15.32856214772949599, 34.49999999999999289 ) ) ;
#12425=CARTESIAN_POINT ( 'NONE',  ( -30.71432649547681137, -21.52377453480933056, 37.50000000000097344 ) ) ;
#12427=CARTESIAN_POINT ( 'NONE',  ( -24.03448224033878944, 8.660042335149839232, 49.47829057475703962 ) ) ;
#12431=B_SPLINE_CURVE_WITH_KNOTS ( 'NONE', 3,
 ( #28888, #24655, #492, #17646, #5790, #960, #786, #3290, #19984, #29033, #22006, #3455, #12972, #29502, #10155, #7670 ),
 .UNSPECIFIED., .F., .F.,
 ( 4, 2, 2, 2, 2, 2, 2, 4 ),
 ( 2.980374332565958659E-07, 0.0009280375596593484246, 0.001391907320772401216, 0.001855777081885454224, 0.002319646842998507232, 0.002783516604111560024, 0.003247386365224613249, 0.003711256126337666040 ),
 .UNSPECIFIED. ) ;
#12457=EDGE_LOOP ( 'NONE', ( #21825, #4123, #15349 ) ) ;
#12473=CARTESIAN_POINT ( 'NONE',  ( 7.628653938386951161, 41.77449438652679703, 28.90251124119662762 ) ) ;
#12477=CARTESIAN_POINT ( 'NONE',  ( -23.60134417525909001, -33.84107530290921062, 29.65494239027400525 ) ) ;
#12510=CARTESIAN_POINT ( 'NONE',  ( 25.22106791543724924, 28.20183085419529334, 34.49999999999999289 ) ) ;
#12512=( BOUNDED_SURFACE ( )  B_SPLINE_SURFACE ( 3, 1, ( 
 ( #3248, #14953 ),
 ( #8101, #12628 ),
 ( #22118, #745 ),
 ( #10265, #12774 ) ),
 .UNSPECIFIED., .F., .F., .F. ) 
 B_SPLINE_SURFACE_WITH_KNOTS ( ( 4, 4 ),
 ( 2, 2 ),
 ( 0.000000000000000000, 1.000000000000000000 ),
 ( 0.000000000000000000, 1.000000000000000000 ),
 .UNSPECIFIED. ) 
 GEOMETRIC_REPRESENTATION_ITEM ( )  RATIONAL_B_SPLINE_SURFACE ( (
 ( 1.000000000000000000, 1.000000000000000000),
 ( 0.3333333333333333703, 0.3333333333333333703),
 ( 0.3333333333333333703, 0.3333333333333333703),
 ( 1.000000000000000000, 1.000000000000000000) ) ) 
 REPRESENTATION_ITEM ( '' )  SURFACE ( )  );
#12525=LINE ( 'NONE', #29047, #19946 ) ;
#12541=CARTESIAN_POINT ( 'NONE',  ( -27.03074382657074182, -6.449748410230987439, 47.21042702067970964 ) ) ;
#12560=VERTEX_POINT ( 'NONE', #27871 ) ;
#12561=VERTEX_POINT ( 'NONE', #25977 ) ;
#12577=CARTESIAN_POINT ( 'NONE',  ( -21.73953648291186269, -30.57930865885014882, 37.49999999997677236 ) ) ;
#12597=ORIENTED_EDGE ( 'NONE', *, *, #20998, .F. ) ;
#12601=EDGE_LOOP ( 'NONE', ( #11353, #5683 ) ) ;
#12603=CARTESIAN_POINT ( 'NONE',  ( -34.24107012425980656, -12.20860444836018388, 27.50000000000000355 ) ) ;
#12616=CARTESIAN_POINT ( 'NONE',  ( 16.55859027208438405, 35.07752759152815258, 27.50000000000000355 ) ) ;
#12619=CARTESIAN_POINT ( 'NONE',  ( 38.44330510386382826, -7.601442456462468300, 32.05526165865716592 ) ) ;
#12626=CARTESIAN_POINT ( 'NONE',  ( -35.09604417355253503, 18.57963138642829293, 31.21515930947347428 ) ) ;
#12628=CARTESIAN_POINT ( 'NONE',  ( 77.99999999999998579, -42.50000000000002132, 27.50000000000000711 ) ) ;
#12633=CARTESIAN_POINT ( 'NONE',  ( 33.18263104983779499, -15.34882887482265090, 34.49999999999998579 ) ) ;
#12645=ORIENTED_EDGE ( 'NONE', *, *, #22971, .T. ) ;
#12659=CARTESIAN_POINT ( 'NONE',  ( -25.07174449839133601, 6.739288358966158299, 44.79593483594015169 ) ) ;
#12664=EDGE_LOOP ( 'NONE', ( #18550, #25345, #4730, #27220, #3873, #16981 ) ) ;
#12665=CARTESIAN_POINT ( 'NONE',  ( 10.02323409478514726, 38.00094089691386046, 34.49999999999999289 ) ) ;
#12670=CARTESIAN_POINT ( 'NONE',  ( -25.41654339919794836, -6.509636863629522097, 48.76343458312125279 ) ) ;
#12672=CARTESIAN_POINT ( 'NONE',  ( -4.163336342344337027E-14, 1.387778780781445676E-14, 52.50000000000000000 ) ) ;
#12678=EDGE_CURVE ( 'NONE', #19313, #20257, #25829, .T. ) ;
#12695=EDGE_LOOP ( 'NONE', ( #10147, #11039, #6694, #21440 ) ) ;
#12698=CARTESIAN_POINT ( 'NONE',  ( -28.99877614713496499, 23.42512202833223256, 34.50000000000000711 ) ) ;
#12728=CARTESIAN_POINT ( 'NONE',  ( -34.05631088549311869, -20.75780206758287605, 34.71020314001439289 ) ) ;
#12752=CARTESIAN_POINT ( 'NONE',  ( -34.89093055204507010, -9.806398194637136356, 27.50000000000000355 ) ) ;
#12760=VERTEX_POINT ( 'NONE', #2890 ) ;
#12767=CARTESIAN_POINT ( 'NONE',  ( 38.99896367101428041, 0.7149996954306816477, 32.23183565673390660 ) ) ;
#12773=CARTESIAN_POINT ( 'NONE',  ( -20.59122450303579299, 36.11886001072432606, 29.42821036418931868 ) ) ;
#12774=CARTESIAN_POINT ( 'NONE',  ( 0.000000000000000000, 42.50000000000000000, 27.50000000000000355 ) ) ;
#12815=CARTESIAN_POINT ( 'NONE',  ( -35.99999999999995026, -1.782879839938830147, 34.75735931288075165 ) ) ;
#12820=CARTESIAN_POINT ( 'NONE',  ( -32.28307784207223108, 8.475829241206282560, 41.62281023987520001 ) ) ;
#12824=CARTESIAN_POINT ( 'NONE',  ( 24.44496207165490631, -7.595930209050163029, 49.40206402021031096 ) ) ;
#12836=CARTESIAN_POINT ( 'NONE',  ( 19.54193581524819479, 36.78865913394601961, 34.51621032707691938 ) ) ;
#12841=CARTESIAN_POINT ( 'NONE',  ( -33.37783937289808733, -9.491076832576640143, 36.05646065681573020 ) ) ;
#12844=ORIENTED_EDGE ( 'NONE', *, *, #6776, .F. ) ;
#12853=CARTESIAN_POINT ( 'NONE',  ( -18.22639394488086140, 34.06491890574931602, 34.50000000000000000 ) ) ;
#12854=DIRECTION ( 'NONE',  ( 1.000000000000000000, 0.000000000000000000, 0.000000000000000000 ) ) ;
#12877=CARTESIAN_POINT ( 'NONE',  ( -32.14097302481091134, 14.40131566728161161, 35.53783135158884221 ) ) ;
#12879=CARTESIAN_POINT ( 'NONE',  ( 1.897190766380719928, -42.45663748335544341, 28.84347297178204528 ) ) ;
#12890=CARTESIAN_POINT ( 'NONE',  ( -39.02782386566561001, 2.105345730448363373, 35.08203289608308495 ) ) ;
#12896=PLANE ( 'NONE',  #10345 ) ;
#12912=VERTEX_POINT ( 'NONE', #27060 ) ;
#12932=ORIENTED_EDGE ( 'NONE', *, *, #18006, .T. ) ;
#12934=CARTESIAN_POINT ( 'NONE',  ( 2.593413279260996074, -42.50000000000001421, 28.83974596215560027 ) ) ;
#12936=AXIS2_PLACEMENT_3D ( 'NONE', #18241, #22908, #4189 ) ;
#12937=DIRECTION ( 'NONE',  ( 0.000000000000000000, 0.000000000000000000, 1.000000000000000000 ) ) ;
#12938=CARTESIAN_POINT ( 'NONE',  ( -34.20814422162067814, -20.42093422158073679, 31.03595515439071306 ) ) ;
#12968=CARTESIAN_POINT ( 'NONE',  ( 33.56327786402390245, 10.22184702512350540, 39.91486591007065954 ) ) ;
#12970=CARTESIAN_POINT ( 'NONE',  ( -4.677126025380957230, 39.24912351428227453, 34.80090346875804386 ) ) ;
#12972=CARTESIAN_POINT ( 'NONE',  ( 31.89119714134807637, 14.79609055705961929, 39.84392849735361608 ) ) ;
#13000=VERTEX_POINT ( 'NONE', #849 ) ;
#13004=EDGE_CURVE ( 'NONE', #4107, #19828, #29516, .T. ) ;
#13013=ORIENTED_EDGE ( 'NONE', *, *, #21930, .F. ) ;
#13023=ORIENTED_EDGE ( 'NONE', *, *, #20259, .F. ) ;
#13034=ORIENTED_EDGE ( 'NONE', *, *, #25344, .F. ) ;
#13037=PLANE ( 'NONE',  #5369 ) ;
#13044=VECTOR ( 'NONE', #17323, 1000.000000000000000 ) ;
#13049=CARTESIAN_POINT ( 'NONE',  ( 31.46019086465473436, 15.19107625323260891, 35.82171084658595817 ) ) ;
#13059=CARTESIAN_POINT ( 'NONE',  ( 32.60608336680204644, -8.625548295239456209, 41.27238065709471471 ) ) ;
#13062=ORIENTED_EDGE ( 'NONE', *, *, #3310, .F. ) ;
#13074=ORIENTED_EDGE ( 'NONE', *, *, #2312, .F. ) ;
#13086=CARTESIAN_POINT ( 'NONE',  ( -27.86235613436986114, 14.72519157938688750, 39.24389099736758624 ) ) ;
#13093=ORIENTED_EDGE ( 'NONE', *, *, #25344, .T. ) ;
#13124=CARTESIAN_POINT ( 'NONE',  ( -32.31576317091163730, 17.59561277345963504, 34.80090346875804386 ) ) ;
#13133=ORIENTED_EDGE ( 'NONE', *, *, #21956, .T. ) ;
#13146=CARTESIAN_POINT ( 'NONE',  ( 32.60829997825918980, 13.18983524832148646, 39.84356070656653515 ) ) ;
#13172=CARTESIAN_POINT ( 'NONE',  ( -30.74201181684193784, 15.50830195949553314, 36.32560960729297506 ) ) ;
#13186=EDGE_CURVE ( 'NONE', #1048, #3168, #12525, .T. ) ;
#13188=CARTESIAN_POINT ( 'NONE',  ( -23.07950435457407679, -11.50806656539752737, 49.21048435262065368 ) ) ;
#13198=CARTESIAN_POINT ( 'NONE',  ( 27.03074382657074537, -6.449748410230991880, -16.55003854064094426 ) ) ;
#13208=CARTESIAN_POINT ( 'NONE',  ( 33.56327786402393087, -10.22184951998668190, 39.91486517541614631 ) ) ;
#13217=VERTEX_POINT ( 'NONE', #654 ) ;
#13226=B_SPLINE_CURVE_WITH_KNOTS ( 'NONE', 3,
 ( #16971, #11995, #19616, #26489, #14942, #26814, #14782, #24452, #5123, #14634, #24135, #131 ),
 .UNSPECIFIED., .F., .F.,
 ( 4, 2, 2, 2, 2, 4 ),
 ( 2.975096543230397156E-07, 0.0009689891193463222828, 0.001937680729038321684, 0.002906372338730320651, 0.003390718143576315364, 0.003875063948422309643 ),
 .UNSPECIFIED. ) ;
#13229=CARTESIAN_POINT ( 'NONE',  ( -11.92482408165411556, 35.57293605924007096, 37.49999999996230571 ) ) ;
#13251=CARTESIAN_POINT ( 'NONE',  ( 28.55068628633582861, -24.19494186940697844, 34.80090346875809360 ) ) ;
#13261=CARTESIAN_POINT ( 'NONE',  ( -24.35970437652574105, 13.37404834226503247, 47.21042702067971675 ) ) ;
#13267=CARTESIAN_POINT ( 'NONE',  ( -33.51229671200703564, -9.872960191568498800, 40.06382167421666907 ) ) ;
#13277=CARTESIAN_POINT ( 'NONE',  ( 33.41082347385297169, 9.568393510027426885, 40.24615645622728266 ) ) ;
#13293=DIRECTION ( 'NONE',  ( -0.000000000000000000, -0.000000000000000000, 1.000000000000000000 ) ) ;
#13304=CARTESIAN_POINT ( 'NONE',  ( -33.56834390605528995, 10.30393839426307423, 39.88609648707288358 ) ) ;
#13308=UNCERTAINTY_MEASURE_WITH_UNIT (LENGTH_MEASURE( 1.000000000000000082E-05 ), #10564, 'distance_accuracy_value', 'NONE');
#13330=CARTESIAN_POINT ( 'NONE',  ( -33.56834390605528995, 10.30393839426307423, 35.64345579995360680 ) ) ;
#13335=CARTESIAN_POINT ( 'NONE',  ( -0.1851967867237511445, -37.50414277995155743, 37.50000000001682565 ) ) ;
#13345=CARTESIAN_POINT ( 'NONE',  ( -23.07950435457408389, -11.74770253185616298, 49.10355149311385503 ) ) ;
#13346=CARTESIAN_POINT ( 'NONE',  ( -11.92114224723059124, -40.47287111344137145, 29.01828771891121761 ) ) ;
#13349=CARTESIAN_POINT ( 'NONE',  ( -26.12638453225885726, -6.310846377660610074, 43.87962907655882105 ) ) ;
#13356=CARTESIAN_POINT ( 'NONE',  ( 31.57476163834522964, 15.10795358447669479, 35.75454235600946618 ) ) ;
#13367=CARTESIAN_POINT ( 'NONE',  ( 35.78336344873347485, -4.414649291701021383, 34.71346399078482392 ) ) ;
#13377=SHAPE_REPRESENTATION_RELATIONSHIP ( 'NONE' , 'NONE' ,  #19685, #23278 ) ;
#13388=ORIENTED_EDGE ( 'NONE', *, *, #9033, .T. ) ;
#13390=EDGE_CURVE ( 'NONE', #5509, #26574, #14498, .T. ) ;
#13415=CARTESIAN_POINT ( 'NONE',  ( 11.52197458429824550, -37.50933785548061650, 27.50000000000000355 ) ) ;
#13437=ORIENTED_EDGE ( 'NONE', *, *, #1025, .F. ) ;
#13448=EDGE_CURVE ( 'NONE', #6144, #23060, #10107, .T. ) ;
#13454=ORIENTED_EDGE ( 'NONE', *, *, #8977, .F. ) ;
#13469=CARTESIAN_POINT ( 'NONE',  ( -32.68301789103641397, 8.668739453992939659, 41.18702913609079985 ) ) ;
#13482=CARTESIAN_POINT ( 'NONE',  ( 32.60829997825920401, -13.18983524832148113, 39.84356070656651383 ) ) ;
#13484=DIRECTION ( 'NONE',  ( -1.000000000000000000, 0.000000000000000000, 0.000000000000000000 ) ) ;
#13487=FACE_OUTER_BOUND ( 'NONE', #13981, .T. ) ;
#13494=CARTESIAN_POINT ( 'NONE',  ( 21.25638073752607227, -35.66179139336605175, 29.47302916183132027 ) ) ;
#13499=EDGE_CURVE ( 'NONE', #18116, #17044, #1563, .T. ) ;
#13503=EDGE_CURVE ( 'NONE', #26303, #3168, #21251, .T. ) ;
#13506=CARTESIAN_POINT ( 'NONE',  ( -13.39580148490130540, -35.10399786391197807, 37.49999999996187228 ) ) ;
#13541=CARTESIAN_POINT ( 'NONE',  ( -4.613788807593795838, 42.22795758926503851, 34.60590817694901489 ) ) ;
#13547=EDGE_LOOP ( 'NONE', ( #26772, #20754, #15697, #23996, #11997, #28388, #10535, #28999, #11533 ) ) ;
#13551=CARTESIAN_POINT ( 'NONE',  ( 17.29228478519430112, -38.19350839570123668, 29.22794746440463243 ) ) ;
#13552=FACE_BOUND ( 'NONE', #6560, .T. ) ;
#13553=CARTESIAN_POINT ( 'NONE',  ( 24.85846090629200233, -6.933313039714898096, 49.19304184080755959 ) ) ;
#13560=CARTESIAN_POINT ( 'NONE',  ( 15.85884089648730289, -35.55173462727349687, 34.80090346875809360 ) ) ;
#13562=ORIENTED_EDGE ( 'NONE', *, *, #17818, .F. ) ;
#13570=CARTESIAN_POINT ( 'NONE',  ( 24.35970437652574105, 13.37404834226503958, 47.21042702067963859 ) ) ;
#13574=CYLINDRICAL_SURFACE ( 'NONE', #4770, 2.000000000000001776 ) ;
#13587=CARTESIAN_POINT ( 'NONE',  ( 32.28307784207223108, 8.475829241206289666, 41.62281023987511475 ) ) ;
#13590=CARTESIAN_POINT ( 'NONE',  ( -35.76481447503397959, 5.202797454133647470, 27.50000000000001066 ) ) ;
#13607=CARTESIAN_POINT ( 'NONE',  ( -23.21352257770656990, 10.78826658734919519, 45.15942333309111234 ) ) ;
#13611=B_SPLINE_CURVE_WITH_KNOTS ( 'NONE', 3,
 ( #29947, #27606, #11215, #18855 ),
 .UNSPECIFIED., .F., .F.,
 ( 4, 4 ),
 ( 3.018024802580205417E-07, 0.007932103453629116285 ),
 .UNSPECIFIED. ) ;
#13648=CARTESIAN_POINT ( 'NONE',  ( 35.05587750292992411, -18.67595856107542218, 34.76255166971075994 ) ) ;
#13656=CARTESIAN_POINT ( 'NONE',  ( -7.734930024145167060, -41.68293636675864633, 34.59191748876874328 ) ) ;
#13667=CARTESIAN_POINT ( 'NONE',  ( -33.42925964089141644, -11.06161099612212695, 39.78814634291941843 ) ) ;
#13679=VECTOR ( 'NONE', #23511, 1000.000000000000000 ) ;
#13700=CYLINDRICAL_SURFACE ( 'NONE', #11310, 1.999999999999998224 ) ;
#13707=CARTESIAN_POINT ( 'NONE',  ( 11.52197458429824550, -37.50933785548061650, 34.80090346875809360 ) ) ;
#13721=DIRECTION ( 'NONE',  ( -0.000000000000000000, -0.000000000000000000, 1.000000000000000000 ) ) ;
#13725=DIRECTION ( 'NONE',  ( -0.000000000000000000, -0.000000000000000000, -1.000000000000000000 ) ) ;
#13728=CARTESIAN_POINT ( 'NONE',  ( -34.13832859401788511, 12.80067323710188276, 27.50000000000001776 ) ) ;
#13743=CARTESIAN_POINT ( 'NONE',  ( -4.163336342344337027E-14, 1.387778780781445676E-14, 37.50000000000000000 ) ) ;
#13768=CARTESIAN_POINT ( 'NONE',  ( -4.163336342344337027E-14, 1.387778780781445676E-14, 51.25735931288069480 ) ) ;
#13770=ADVANCED_FACE ( 'NONE', ( #24093, #2743, #2898 ), #13918, .T. ) ;
#13787=CARTESIAN_POINT ( 'NONE',  ( 16.30589577393280720, -38.63578930953848101, 34.53468016319318679 ) ) ;
#13789=EDGE_LOOP ( 'NONE', ( #7852, #18078, #23903, #14128 ) ) ;
#13798=CARTESIAN_POINT ( 'NONE',  ( -24.75988009833579540, -7.043597625963918141, 45.01551998635112994 ) ) ;
#13809=LINE ( 'NONE', #30626, #3796 ) ;
#13836=DIRECTION ( 'NONE',  ( -0.000000000000000000, -0.000000000000000000, -1.000000000000000000 ) ) ;
#13840=CARTESIAN_POINT ( 'NONE',  ( 1.874238930957292881, 37.52724763749905179, 37.50000000023297986 ) ) ;
#13851=DIRECTION ( 'NONE',  ( 1.000000000000000000, 0.000000000000000000, 0.000000000000000000 ) ) ;
#13852=CARTESIAN_POINT ( 'NONE',  ( 24.44496207165490276, 7.595930209050162141, 49.40206402021032517 ) ) ;
#13859=CARTESIAN_POINT ( 'NONE',  ( 32.31576317091162309, 17.59561277345964214, 34.80090346875808649 ) ) ;
#13861=ORIENTED_EDGE ( 'NONE', *, *, #18130, .F. ) ;
#13866=DIRECTION ( 'NONE',  ( -0.000000000000000000, -0.000000000000000000, 1.000000000000000000 ) ) ;
#13867=CARTESIAN_POINT ( 'NONE',  ( 23.07491035053308437, 11.55692089822198376, 49.19304184087432219 ) ) ;
#13874=CARTESIAN_POINT ( 'NONE',  ( 32.19782014694308003, -14.25394737442115201, -16.55003854064094426 ) ) ;
#13876=VERTEX_POINT ( 'NONE', #17696 ) ;
#13882=CARTESIAN_POINT ( 'NONE',  ( -34.13832859401785669, -12.80067323710187921, 34.80090346875803675 ) ) ;
#13896=CIRCLE ( 'NONE', #14896, 36.25735931288072322 ) ;
#13898=CARTESIAN_POINT ( 'NONE',  ( 24.35970437652574816, -13.37404834226503958, 42.96778633356033339 ) ) ;
#13907=ORIENTED_EDGE ( 'NONE', *, *, #20420, .T. ) ;
#13913=CARTESIAN_POINT ( 'NONE',  ( 35.72891310271008081, 4.992827801344182248, 27.50000000000001066 ) ) ;
#13918=CONICAL_SURFACE ( 'NONE', #7943, 37.50000000000001421, 0.7853981633974500554 ) ;
#13927=CARTESIAN_POINT ( 'NONE',  ( -23.21352257770656990, -10.78826658734919519, 49.40206402021038201 ) ) ;
#13935=CARTESIAN_POINT ( 'NONE',  ( 32.23417439153795527, -24.08006005343069944, 30.66707834874007332 ) ) ;
#13936=EDGE_CURVE ( 'NONE', #29313, #12760, #29459, .T. ) ;
#13937=FACE_OUTER_BOUND ( 'NONE', #9255, .T. ) ;
#13939=CARTESIAN_POINT ( 'NONE',  ( 23.21352257770656635, -10.78826658734920052, 49.40206402021031806 ) ) ;
#13940=DIRECTION ( 'NONE',  ( -0.9329908884337534403, -0.3598999890241668664, 0.000000000000000000 ) ) ;
#13947=CARTESIAN_POINT ( 'NONE',  ( -30.86161751192252467, -15.46691422980912733, 40.47962024281694937 ) ) ;
#13965=CARTESIAN_POINT ( 'NONE',  ( -24.02386986937633395, 13.21681873352653902, 43.33784216537009826 ) ) ;
#13968=CARTESIAN_POINT ( 'NONE',  ( 33.56327786402394509, -10.57885966092500851, 35.56709683732771055 ) ) ;
#13981=EDGE_LOOP ( 'NONE', ( #22654, #21133, #10088, #16825 ) ) ;
#13986=CARTESIAN_POINT ( 'NONE',  ( -24.78335882923826006, 28.14977597724353231, 37.50000000000454037 ) ) ;
#13996=CARTESIAN_POINT ( 'NONE',  ( 30.33183837007556249, -13.53414739637283226, -16.55003854064094426 ) ) ;
#14011=DIRECTION ( 'NONE',  ( 1.000000000000000000, 0.000000000000000000, 0.000000000000000000 ) ) ;
#14013=VERTEX_POINT ( 'NONE', #28135 ) ;
#14021=VERTEX_POINT ( 'NONE', #13939 ) ;
#14051=CARTESIAN_POINT ( 'NONE',  ( 30.05895891365310391, -21.74113609263913105, 27.50000000000000000 ) ) ;
#14058=CARTESIAN_POINT ( 'NONE',  ( -30.50257113119997499, 15.54031451041691092, 40.76699977199277214 ) ) ;
#14073=CARTESIAN_POINT ( 'NONE',  ( 14.12697113674015448, -34.75723440155685751, 37.49999999999971578 ) ) ;
#14082=CARTESIAN_POINT ( 'NONE',  ( -32.06725342158289038, -14.54034564589948708, 35.54788606881766810 ) ) ;
#14083=EDGE_LOOP ( 'NONE', ( #28365, #9570, #5473, #26910 ) ) ;
#14093=CARTESIAN_POINT ( 'NONE',  ( 27.03074382657074537, 6.449748410230989215, 42.96778633356034760 ) ) ;
#14094=ORIENTED_EDGE ( 'NONE', *, *, #13936, .T. ) ;
#14103=CARTESIAN_POINT ( 'NONE',  ( 5.060094141397912360, 42.14075867279367316, 28.87075318537527835 ) ) ;
#14111=ORIENTED_EDGE ( 'NONE', *, *, #22309, .T. ) ;
#14123=CARTESIAN_POINT ( 'NONE',  ( -15.22124877282432465, 34.27704336327021650, 37.50000000002827250 ) ) ;
#14128=ORIENTED_EDGE ( 'NONE', *, *, #3316, .F. ) ;
#14138=LINE ( 'NONE', #4324, #29707 ) ;
#14167=FACE_OUTER_BOUND ( 'NONE', #2157, .T. ) ;
#14171=CARTESIAN_POINT ( 'NONE',  ( -23.09047454507859953, 11.74540567832116267, 49.09408197974163812 ) ) ;
#14186=CARTESIAN_POINT ( 'NONE',  ( -2.492600117579355956, -39.42873062461828226, 27.50000000000000355 ) ) ;
#14201=CARTESIAN_POINT ( 'NONE',  ( 34.43169391940249113, -11.54542193137334394, 27.50000000000000355 ) ) ;
#14206=CARTESIAN_POINT ( 'NONE',  ( -30.74201181684194850, 15.50830195949553669, 40.56825029441224473 ) ) ;
#14222=CARTESIAN_POINT ( 'NONE',  ( 27.16566537401950043, 25.85840940979817049, 37.50000000000431299 ) ) ;
#14237=ORIENTED_EDGE ( 'NONE', *, *, #24407, .F. ) ;
#14258=CARTESIAN_POINT ( 'NONE',  ( 32.19782014694308003, -14.25394737442115201, 35.54550565580006349 ) ) ;
#14272=CARTESIAN_POINT ( 'NONE',  ( -26.07963561311912670, 31.61094817644626076, 34.51864978005331608 ) ) ;
#14327=EDGE_CURVE ( 'NONE', #14013, #11387, #12330, .T. ) ;
#14332=CARTESIAN_POINT ( 'NONE',  ( -24.35970437652574105, 13.37404834226503247, 47.21042702067971675 ) ) ;
#14336=CARTESIAN_POINT ( 'NONE',  ( 23.21352257770656635, -10.78826658734920052, 45.15942333309103418 ) ) ;
#14339=CYLINDRICAL_SURFACE ( 'NONE', #4339, 2.000000000000005329 ) ;
#14348=CARTESIAN_POINT ( 'NONE',  ( -19.70185583149091002, -33.06308933231057523, 27.50000000000000355 ) ) ;
#14349=EDGE_CURVE ( 'NONE', #254, #19220, #6738, .T. ) ;
#14355=CARTESIAN_POINT ( 'NONE',  ( -5.095241848980792021, -39.11820605553161556, 34.50000000000000000 ) ) ;
#14369=CARTESIAN_POINT ( 'NONE',  ( 23.90632052215872605, 29.53616140628007614, 27.50000000000000355 ) ) ;
#14371=CARTESIAN_POINT ( 'NONE',  ( -24.44496207165490276, -7.595930209050158588, 49.40206402021039622 ) ) ;
#14389=EDGE_CURVE ( 'NONE', #10056, #165, #22938, .T. ) ;
#14394=CARTESIAN_POINT ( 'NONE',  ( 38.97083381611543729, -2.113745753963891083, 35.07647338176046503 ) ) ;
#14405=CARTESIAN_POINT ( 'NONE',  ( -29.81956388892670518, -15.48018185647901213, 37.15911814917528488 ) ) ;
#14413=CARTESIAN_POINT ( 'NONE',  ( 0.000000000000000000, 39.50000000000000000, 27.50000000000000355 ) ) ;
#14421=CARTESIAN_POINT ( 'NONE',  ( 30.53339558441486190, 7.800891647352844238, 39.24389099736750808 ) ) ;
#14447=CARTESIAN_POINT ( 'NONE',  ( -34.55463468735881349, 14.62320705866887494, 37.50000000001273293 ) ) ;
#14450=CARTESIAN_POINT ( 'NONE',  ( 33.41082347385297169, 9.568393510027430438, 36.00351576910800588 ) ) ;
#14452=VERTEX_POINT ( 'NONE', #28086 ) ;
#14471=ADVANCED_FACE ( 'NONE', ( #6102 ), #25130, .F. ) ;
#14485=CARTESIAN_POINT ( 'NONE',  ( -23.12946144662537051, 11.96621729904739517, 48.95860290871405596 ) ) ;
#14498=( BOUNDED_CURVE ( )  B_SPLINE_CURVE ( 3, ( #8477, #975, #22336, #17506 ),
 .UNSPECIFIED., .F., .T. ) 
 B_SPLINE_CURVE_WITH_KNOTS ( ( 4, 4 ),
 ( 3.141592653589793116, 6.283185307179586232 ),
 .UNSPECIFIED. ) 
 CURVE ( )  GEOMETRIC_REPRESENTATION_ITEM ( )  RATIONAL_B_SPLINE_CURVE ( ( 1.000000000000000000, 0.3333333333333333703, 0.3333333333333333703, 1.000000000000000000 ) ) 
 REPRESENTATION_ITEM ( '' )  );
#14506=CARTESIAN_POINT ( 'NONE',  ( -31.59044894475038134, -19.10522403758187338, 27.50000000000000355 ) ) ;
#14510=CARTESIAN_POINT ( 'NONE',  ( -13.83774706505031560, -36.52929077895569066, 34.49999999999999289 ) ) ;
#14511=ADVANCED_FACE ( 'NONE', ( #30569, #2333 ), #4527, .F. ) ;
#14513=FACE_OUTER_BOUND ( 'NONE', #28409, .T. ) ;
#14521=DIRECTION ( 'NONE',  ( 0.9329908884337542174, -0.3598999890241650901, 0.000000000000000000 ) ) ;
#14528=CARTESIAN_POINT ( 'NONE',  ( 33.42925964089141644, -11.06161099612213228, 39.78814634291933316 ) ) ;
#14548=CARTESIAN_POINT ( 'NONE',  ( 36.66051849534079565, 8.298796628992828772, 37.50000000001189449 ) ) ;
#14554=LINE ( 'NONE', #24050, #27669 ) ;
#14556=ORIENTED_EDGE ( 'NONE', *, *, #3915, .F. ) ;
#14597=CARTESIAN_POINT ( 'NONE',  ( -18.39976944410068072, 37.47990255558614336, 29.29674481779093043 ) ) ;
#14603=CARTESIAN_POINT ( 'NONE',  ( 33.03707461445869598, 8.975870916883787132, 36.52286458921579992 ) ) ;
#14611=CARTESIAN_POINT ( 'NONE',  ( -77.99999999999998579, -42.49999999999998579, 27.50000000000000711 ) ) ;
#14617=AXIS2_PLACEMENT_3D ( 'NONE', #3331, #24689, #10195 ) ;
#14634=CARTESIAN_POINT ( 'NONE',  ( 23.11524226670866611, -11.10088790631999345, 45.11515778357083661 ) ) ;
#14638=CARTESIAN_POINT ( 'NONE',  ( 32.19782014694308003, -14.25394737442115201, 39.78814634291934738 ) ) ;
#14642=FACE_OUTER_BOUND ( 'NONE', #12695, .T. ) ;
#14659=CARTESIAN_POINT ( 'NONE',  ( -29.01070392382221286, -23.40766234503086807, 34.49999999999998579 ) ) ;
#14672=CARTESIAN_POINT ( 'NONE',  ( 33.56327786402390245, 10.34181101807379655, -16.55003854064094426 ) ) ;
#14690=CARTESIAN_POINT ( 'NONE',  ( 38.70786393739909670, 5.827369745586353567, 35.04830057171592728 ) ) ;
#14697=ORIENTED_EDGE ( 'NONE', *, *, #26732, .F. ) ;
#14724=CARTESIAN_POINT ( 'NONE',  ( -23.26375789455195786, 12.37328455203049771, 44.40817556379787590 ) ) ;
#14741=CARTESIAN_POINT ( 'NONE',  ( -37.58583663907551653, -0.5225704585679834535, 37.50000000000396483 ) ) ;
#14745=CARTESIAN_POINT ( 'NONE',  ( 33.55239377822428537, 10.10392708029668363, 35.71678343307738146 ) ) ;
#14746=FACE_BOUND ( 'NONE', #10568, .T. ) ;
#14754=CARTESIAN_POINT ( 'NONE',  ( -77.99999999999998579, 42.50000000000000000, 27.50000000000000711 ) ) ;
#14764=AXIS2_PLACEMENT_3D ( 'NONE', #26472, #29120, #7757 ) ;
#14779=AXIS2_PLACEMENT_3D ( 'NONE', #18499, #11475, #28000 ) ;
#14782=CARTESIAN_POINT ( 'NONE',  ( 23.11727550875142612, -11.99039815441031465, 44.71664046407185822 ) ) ;
#14795=EDGE_LOOP ( 'NONE', ( #16165, #13133, #2463, #30250 ) ) ;
#14801=EDGE_LOOP ( 'NONE', ( #28343, #21446, #18407, #16189, #30212, #2566, #12645, #16294, #11437 ) ) ;
#14802=ORIENTED_EDGE ( 'NONE', *, *, #13503, .T. ) ;
#14805=B_SPLINE_CURVE_WITH_KNOTS ( 'NONE', 3,
 ( #1307, #29865, #4712, #13927 ),
 .UNSPECIFIED., .F., .F.,
 ( 4, 4 ),
 ( 2.143643656977390230E-07, 0.003421830178490235883 ),
 .UNSPECIFIED. ) ;
#14830=CARTESIAN_POINT ( 'NONE',  ( 19.13430944348616691, 33.52606101487586443, 34.49999999999999289 ) ) ;
#14849=CARTESIAN_POINT ( 'NONE',  ( 14.39597666885513050, 39.52646374787653372, 29.10435809556016551 ) ) ;
#14854=VECTOR ( 'NONE', #15162, 1000.000000000000000 ) ;
#14872=CARTESIAN_POINT ( 'NONE',  ( 24.35970437652574105, 13.37404834226503958, 42.96778633356035471 ) ) ;
#14890=CARTESIAN_POINT ( 'NONE',  ( 33.56327786402390245, 10.34181101807379299, 39.87954049117193023 ) ) ;
#14896=AXIS2_PLACEMENT_3D ( 'NONE', #9281, #30348, #4602 ) ;
#14905=CARTESIAN_POINT ( 'NONE',  ( -25.40309444575802900, -32.28060097791307470, 34.51338776223392557 ) ) ;
#14929=CARTESIAN_POINT ( 'NONE',  ( -31.56327786402390245, 10.34181101807378944, -16.55003854064094426 ) ) ;
#14942=CARTESIAN_POINT ( 'NONE',  ( 23.44182307864140569, -12.68276878097691807, 44.10491087720090064 ) ) ;
#14944=CARTESIAN_POINT ( 'NONE',  ( 33.89076711745516235, -13.33308044341245768, 27.49999999999999645 ) ) ;
#14947=CARTESIAN_POINT ( 'NONE',  ( 33.36352722101803892, 22.16012013285964599, 30.86670504923349512 ) ) ;
#14952=CARTESIAN_POINT ( 'NONE',  ( -31.99717184760054423, -24.33433105396149543, 30.64030087745031850 ) ) ;
#14953=CARTESIAN_POINT ( 'NONE',  ( -4.776122516674677878E-15, -42.50000000000000000, 27.50000000000000355 ) ) ;
#14957=CARTESIAN_POINT ( 'NONE',  ( 29.54399056023980918, -22.57198099544491754, 34.49999999999999289 ) ) ;
#14974=EDGE_LOOP ( 'NONE', ( #18058, #30595, #15255, #3949 ) ) ;
#14976=CARTESIAN_POINT ( 'NONE',  ( 30.50257113119998564, -15.54031451041691447, 36.52435908487338168 ) ) ;
#14983=CARTESIAN_POINT ( 'NONE',  ( 0.000000000000000000, 39.50000000000000000, 34.49999999999999289 ) ) ;
#14986=CARTESIAN_POINT ( 'NONE',  ( -15.85884089648730999, 35.55173462727350397, 34.80090346875804386 ) ) ;
#14990=CARTESIAN_POINT ( 'NONE',  ( -27.03074382657074182, -6.449748410230987439, 47.21042702067970964 ) ) ;
#15015=DIRECTION ( 'NONE',  ( 1.000000000000000000, 0.000000000000000000, 0.000000000000000000 ) ) ;
#15035=CARTESIAN_POINT ( 'NONE',  ( 1.577737821089430392, -37.47138393967439640, 37.49999999998041744 ) ) ;
#15045=CARTESIAN_POINT ( 'NONE',  ( -19.50000000000000711, 1.046363422724301872E-14, 51.25735931288069480 ) ) ;
#15047=CARTESIAN_POINT ( 'NONE',  ( -38.24313799765437949, -8.361081211805744928, 35.00208094606055909 ) ) ;
#15063=CARTESIAN_POINT ( 'NONE',  ( -77.99999999999998579, 42.50000000000000711, 32.33822642395377045 ) ) ;
#15074=CARTESIAN_POINT ( 'NONE',  ( -26.83887921667331966, -26.32914559372739660, 27.50000000000000000 ) ) ;
#15084=ADVANCED_FACE ( 'NONE', ( #15214 ), #19754, .F. ) ;
#15097=CARTESIAN_POINT ( 'NONE',  ( -38.99591598333270781, -2.632255423871425304, 32.22937204864898320 ) ) ;
#15109=CARTESIAN_POINT ( 'NONE',  ( 33.01877980957529957, 12.12572312222181026, 35.60092001944724416 ) ) ;
#15126=ORIENTED_EDGE ( 'NONE', *, *, #26946, .F. ) ;
#15130=CARTESIAN_POINT ( 'NONE',  ( 31.22647667302026520, -15.32805873036034860, 35.97188228574909630 ) ) ;
#15135=CARTESIAN_POINT ( 'NONE',  ( 20.76278282699725608, 32.33563723208181528, 34.49999999999999289 ) ) ;
#15142=CARTESIAN_POINT ( 'NONE',  ( 24.03448224033878944, -8.660042335149841009, 49.47829057475696857 ) ) ;
#15144=CIRCLE ( 'NONE', #11177, 22.49999999999996447 ) ;
#15150=CARTESIAN_POINT ( 'NONE',  ( 19.27189572260205708, 36.95578567799407921, 29.34714106128156885 ) ) ;
#15162=DIRECTION ( 'NONE',  ( -0.000000000000000000, -0.000000000000000000, 1.000000000000000000 ) ) ;
#15178=CARTESIAN_POINT ( 'NONE',  ( 33.56327786402390245, -10.34181101807379477, 35.63689980405263924 ) ) ;
#15181=CARTESIAN_POINT ( 'NONE',  ( -32.19782014694307293, 14.25394737442115733, 35.54550565580015586 ) ) ;
#15183=CARTESIAN_POINT ( 'NONE',  ( -5.127072262013855131, -42.13114360820154047, 28.87158698979397897 ) ) ;
#15192=CARTESIAN_POINT ( 'NONE',  ( -38.38780269126310429, -7.528505152340548179, 32.04353250950420318 ) ) ;
#15214=FACE_OUTER_BOUND ( 'NONE', #20347, .T. ) ;
#15216=CARTESIAN_POINT ( 'NONE',  ( -4.962407341831601038, -39.12863361840854282, 27.50000000000000000 ) ) ;
#15231=EDGE_CURVE ( 'NONE', #5196, #20389, #9601, .T. ) ;
#15239=CARTESIAN_POINT ( 'NONE',  ( 6.601643239663004076E-16, 42.50000000000000000, 28.83974596215562514 ) ) ;
#15255=ORIENTED_EDGE ( 'NONE', *, *, #12246, .T. ) ;
#15284=AXIS2_PLACEMENT_3D ( 'NONE', #12672, #22166, #29357 ) ;
#15300=CARTESIAN_POINT ( 'NONE',  ( -23.72453467988983178, -12.99099554674205947, 47.95154756196049561 ) ) ;
#15309=CARTESIAN_POINT ( 'NONE',  ( 24.50428919468314959, 7.442132857256930301, 45.14840622132430781 ) ) ;
#15311=CARTESIAN_POINT ( 'NONE',  ( -33.52485258639264032, 10.76172163581451713, 39.79052675593855781 ) ) ;
#15319=ORIENTED_EDGE ( 'NONE', *, *, #29197, .F. ) ;
#15349=ORIENTED_EDGE ( 'NONE', *, *, #17671, .F. ) ;
#15354=B_SPLINE_SURFACE_WITH_KNOTS ( 'NONE', 3, 1, ( 
 ( #20414, #18229 ),
 ( #4333, #28042 ),
 ( #27906, #4180 ),
 ( #30391, #25243 ),
 ( #13707, #13415 ),
 ( #13560, #3890 ),
 ( #1848, #15572 ),
 ( #3735, #6672 ),
 ( #23039, #27750 ),
 ( #18402, #11206 ),
 ( #13251, #25409 ),
 ( #8421, #25092 ),
 ( #6529, #16041 ),
 ( #20866, #9028 ),
 ( #8716, #18541 ),
 ( #22740, #25553 ),
 ( #1398, #22898 ),
 ( #25703, #8878 ),
 ( #15725, #20703 ),
 ( #4033, #16187 ),
 ( #6381, #6219 ),
 ( #13859, #23360 ),
 ( #29781, #15896 ),
 ( #10912, #10744 ),
 ( #20256, #17932 ),
 ( #8574, #30232 ),
 ( #18077, #27597 ),
 ( #1545, #11056 ),
 ( #20556, #30081 ),
 ( #2146, #23648 ),
 ( #16349, #2462 ),
 ( #4952, #25864 ),
 ( #26473, #16955 ),
 ( #18846, #23504 ) ),
 .UNSPECIFIED., .F., .F., .F.,
 ( 4, 2, 2, 2, 2, 2, 2, 2, 2, 2, 2, 2, 2, 2, 2, 2, 4 ),
 ( 2, 2 ),
 ( 0.000000000000000000, 0.06249999999999998612, 0.1249999999999999722, 0.1874999999999999445, 0.2499999999999999445, 0.3125000000000000000, 0.3750000000000000000, 0.4375000000000000000, 0.5000000000000000000, 0.5625000000000001110, 0.6250000000000001110, 0.6875000000000001110, 0.7500000000000000000, 0.8125000000000000000, 0.8750000000000000000, 0.9375000000000000000, 1.000000000000000000 ),
 ( 0.000000000000000000, 1.000000000000000000 ),
 .UNSPECIFIED. ) ;
#15357=DIRECTION ( 'NONE',  ( -0.000000000000000000, -0.000000000000000000, 1.000000000000000000 ) ) ;
#15358=CARTESIAN_POINT ( 'NONE',  ( -38.81367831590564066, -4.342395794384154684, 32.17324057660533043 ) ) ;
#15375=( GEOMETRIC_REPRESENTATION_CONTEXT ( 3 ) GLOBAL_UNCERTAINTY_ASSIGNED_CONTEXT ( ( #13308 ) ) GLOBAL_UNIT_ASSIGNED_CONTEXT ( ( #10564, #30201, #6344 ) ) REPRESENTATION_CONTEXT ( 'NONE', 'WORKASPACE' ) );
#15402=CARTESIAN_POINT ( 'NONE',  ( 23.63378365164496486, -33.81425525858435321, 29.65764705046944982 ) ) ;
#15432=ORIENTED_EDGE ( 'NONE', *, *, #5741, .F. ) ;
#15434=CARTESIAN_POINT ( 'NONE',  ( 30.03865005752671991, -15.52610542268209848, 36.94359686637162099 ) ) ;
#15464=EDGE_CURVE ( 'NONE', #23060, #4164, #25936, .T. ) ;
#15467=CARTESIAN_POINT ( 'NONE',  ( -32.28307784207223108, -8.475829241206282560, 37.38016955275590902 ) ) ;
#15520=AXIS2_PLACEMENT_3D ( 'NONE', #2667, #14521, #25074 ) ;
#15524=CARTESIAN_POINT ( 'NONE',  ( 24.14277784031759566, 13.29036922066994642, 43.19821070588412226 ) ) ;
#15553=CARTESIAN_POINT ( 'NONE',  ( -12.58753388439931165, 40.25309894602420258, 34.56092818870066452 ) ) ;
#15558=LINE ( 'NONE', #776, #13044 ) ;
#15572=CARTESIAN_POINT ( 'NONE',  ( 17.94248964168179583, -34.33858135081684537, 27.49999999999999645 ) ) ;
#15583=CARTESIAN_POINT ( 'NONE',  ( -29.61203839202723032, 15.40012917324033204, 41.62281023987520001 ) ) ;
#15586=FACE_OUTER_BOUND ( 'NONE', #1963, .T. ) ;
#15601=CARTESIAN_POINT ( 'NONE',  ( -15.85884089648730644, -35.55173462727348266, 34.80090346875803675 ) ) ;
#15621=B_SPLINE_CURVE_WITH_KNOTS ( 'NONE', 3,
 ( #25898, #4683, #4529, #6572, #21192, #13607 ),
 .UNSPECIFIED., .F., .F.,
 ( 4, 2, 4 ),
 ( 0.003121276445852156928, 0.003498170197137229383, 0.003875063948422301837 ),
 .UNSPECIFIED. ) ;
#15649=CARTESIAN_POINT ( 'NONE',  ( -33.51206231511395117, 9.871883628028006896, 35.82171084650917692 ) ) ;
#15652=CARTESIAN_POINT ( 'NONE',  ( -29.81954908927653136, 15.48017614753372051, 37.15913391342354544 ) ) ;
#15665=CARTESIAN_POINT ( 'NONE',  ( -9.920192004040607969, -41.10915752540522305, 28.96131254832305757 ) ) ;
#15669=EDGE_CURVE ( 'NONE', #17963, #18819, #10917, .T. ) ;
#15676=CARTESIAN_POINT ( 'NONE',  ( 32.14095006730908466, 14.40137518142634399, 35.53782825234915066 ) ) ;
#15684=CARTESIAN_POINT ( 'NONE',  ( 35.46011056729525279, -7.038057716375242023, 34.64849135038199535 ) ) ;
#15697=ORIENTED_EDGE ( 'NONE', *, *, #16607, .T. ) ;
#15699=B_SPLINE_CURVE_WITH_KNOTS ( 'NONE', 3,
 ( #18132, #22637, #13469, #8314, #1604, #6267, #27346, #17829, #27495, #5971, #20465, #13304, #29843, #15311, #1288, #1455 ),
 .UNSPECIFIED., .F., .F.,
 ( 4, 2, 2, 2, 2, 2, 2, 4 ),
 ( 2.980251112119010967E-07, 0.0009280375473568674505, 0.001391907308479688144, 0.001855777069602508947, 0.002319646830725329966, 0.002783516591848150552, 0.003247386352970971137, 0.003711256114093792156 ),
 .UNSPECIFIED. ) ;
#15701=CARTESIAN_POINT ( 'NONE',  ( -30.74147208807243814, -15.49548351932574697, 36.33144972441046150 ) ) ;
#15703=CARTESIAN_POINT ( 'NONE',  ( -16.58443505991521150, 38.47295314005269518, 29.20253828648597505 ) ) ;
#15709=CARTESIAN_POINT ( 'NONE',  ( 27.03074382657074537, -6.449748410230991880, 47.21042702067962438 ) ) ;
#15713=CARTESIAN_POINT ( 'NONE',  ( 10.13012925513353579, -41.06507652560424049, 28.96509805317834463 ) ) ;
#15722=ADVANCED_FACE ( 'NONE', ( #25710 ), #4340, .F. ) ;
#15725=CARTESIAN_POINT ( 'NONE',  ( 35.76481447503399380, 5.202797454133643917, 34.80090346875810070 ) ) ;
#15729=CARTESIAN_POINT ( 'NONE',  ( -27.03074382657074537, 6.449748410230988327, -16.55003854064094426 ) ) ;
#15732=ORIENTED_EDGE ( 'NONE', *, *, #6683, .T. ) ;
#15736=FACE_OUTER_BOUND ( 'NONE', #14974, .T. ) ;
#15755=CARTESIAN_POINT ( 'NONE',  ( -2.338573377552017440, -39.49999999999999289, 27.49999999999999645 ) ) ;
#15760=B_SPLINE_CURVE_WITH_KNOTS ( 'NONE', 3,
 ( #18649, #28154, #13965, #2102, #4910, #26596, #14724, #24232, #16755, #17651, #8145, #27169 ),
 .UNSPECIFIED., .F., .F.,
 ( 4, 2, 2, 2, 2, 4 ),
 ( 2.975096543306551241E-07, 0.0007805422437037919103, 0.001560786977753253132, 0.002341031711802714355, 0.002731154078827435425, 0.003121276445852156928 ),
 .UNSPECIFIED. ) ;
#15774=CARTESIAN_POINT ( 'NONE',  ( -27.61994877245214397, 25.33817162612066554, 27.50000000000000000 ) ) ;
#15813=CARTESIAN_POINT ( 'NONE',  ( 23.10194695014233091, -34.27363447027268961, 34.50719889637104387 ) ) ;
#15816=VERTEX_POINT ( 'NONE', #2007 ) ;
#15827=CARTESIAN_POINT ( 'NONE',  ( -31.46019086465472725, -15.19107625323260180, 40.06435153370532021 ) ) ;
#15830=CARTESIAN_POINT ( 'NONE',  ( 31.79271162922634630, -14.90794587988476927, 39.88583012296468411 ) ) ;
#15859=EDGE_CURVE ( 'NONE', #5082, #5196, #15144, .T. ) ;
#15866=CARTESIAN_POINT ( 'NONE',  ( -30.86161751192252467, -15.46691422980912733, 36.23697955569767970 ) ) ;
#15878=CARTESIAN_POINT ( 'NONE',  ( 24.50429677314015109, -7.442113211156457631, 45.14840481399649974 ) ) ;
#15880=EDGE_CURVE ( 'NONE', #26848, #11554, #21480, .T. ) ;
#15893=ADVANCED_FACE ( 'NONE', ( #18690 ), #25870, .F. ) ;
#15896=CARTESIAN_POINT ( 'NONE',  ( 31.18890335284658022, 19.89223002944920538, 27.50000000000001066 ) ) ;
#15899=DIRECTION ( 'NONE',  ( -0.3598999890241659783, -0.9329908884337537733, 0.000000000000000000 ) ) ;
#15908=ORIENTED_EDGE ( 'NONE', *, *, #23326, .T. ) ;
#15923=CARTESIAN_POINT ( 'NONE',  ( 32.90011853910910844, 8.843064278303863546, 40.93222828939945401 ) ) ;
#15930=CARTESIAN_POINT ( 'NONE',  ( 29.61203839202725518, -15.40012917324033381, -16.55003854064094426 ) ) ;
#15943=CARTESIAN_POINT ( 'NONE',  ( 23.07593096178834102, -11.40900259639455072, 49.25816067352246108 ) ) ;
#15960=CARTESIAN_POINT ( 'NONE',  ( 33.42925964089141644, -11.06161099612213228, 39.78814634291933316 ) ) ;
#15962=CARTESIAN_POINT ( 'NONE',  ( -31.89304216768362110, 14.79375299452194881, 39.84323675255983943 ) ) ;
#15973=CARTESIAN_POINT ( 'NONE',  ( 20.46113952635996469, -31.44909971395763648, 37.49999999997999112 ) ) ;
#15981=B_SPLINE_CURVE_WITH_KNOTS ( 'NONE', 3,
 ( #27019, #5647, #15142, #12824 ),
 .UNSPECIFIED., .F., .F.,
 ( 4, 4 ),
 ( 2.143643656977389965E-07, 0.003421830178490238485 ),
 .UNSPECIFIED. ) ;
#15983=CARTESIAN_POINT ( 'NONE',  ( -17.87976126528057108, -37.88093910584518653, 34.52266824050962413 ) ) ;
#15985=CARTESIAN_POINT ( 'NONE',  ( -29.81956388892671583, -15.48018185647901213, 41.40175883629457587 ) ) ;
#15986=DIRECTION ( 'NONE',  ( 0.9329908884337542174, 0.3598999890241650901, 0.000000000000000000 ) ) ;
#15992=CARTESIAN_POINT ( 'NONE',  ( -23.07950435457407679, -11.50806656539752737, 49.21048435262065368 ) ) ;
#16041=CARTESIAN_POINT ( 'NONE',  ( 32.31576317091161599, -17.59561277345965280, 27.50000000000000355 ) ) ;
#16056=LINE ( 'NONE', #1704, #16819 ) ;
#16068=VECTOR ( 'NONE', #18409, 1000.000000000000000 ) ;
#16086=CARTESIAN_POINT ( 'NONE',  ( -13.22604046949001066, 36.76012593405532414, 27.49999999999999645 ) ) ;
#16102=ORIENTED_EDGE ( 'NONE', *, *, #551, .T. ) ;
#16107=CARTESIAN_POINT ( 'NONE',  ( -33.01877980957529957, 12.12572312222180493, 35.60092001944732942 ) ) ;
#16125=CARTESIAN_POINT ( 'NONE',  ( 11.91353211314439164, -35.56214078857726690, 37.49999999998971134 ) ) ;
#16134=CARTESIAN_POINT ( 'NONE',  ( -21.24416681158189135, -35.65075532067091757, 34.51006995843407310 ) ) ;
#16136=CARTESIAN_POINT ( 'NONE',  ( -25.88640477275121654, -6.345529225273950580, 44.10491087709822011 ) ) ;
#16142=CARTESIAN_POINT ( 'NONE',  ( 23.07491035053308437, 11.55692089822198554, 44.95040115375503120 ) ) ;
#16152=CARTESIAN_POINT ( 'NONE',  ( 4.221020697412598999, 42.26040651453248387, 28.86037875636509398 ) ) ;
#16165=ORIENTED_EDGE ( 'NONE', *, *, #15880, .F. ) ;
#16173=CARTESIAN_POINT ( 'NONE',  ( -25.88604317058895177, 6.345278376181627600, 44.10533075955778770 ) ) ;
#16180=FACE_BOUND ( 'NONE', #3858, .T. ) ;
#16185=ORIENTED_EDGE ( 'NONE', *, *, #5594, .F. ) ;
#16187=CARTESIAN_POINT ( 'NONE',  ( 34.83396020575241891, 10.30249279383515848, 27.50000000000001066 ) ) ;
#16189=ORIENTED_EDGE ( 'NONE', *, *, #27747, .T. ) ;
#16195=AXIS2_PLACEMENT_3D ( 'NONE', #21374, #25613, #21199 ) ;
#16196=CYLINDRICAL_SURFACE ( 'NONE', #25881, 22.49999999999996447 ) ;
#16198=FACE_OUTER_BOUND ( 'NONE', #2468, .T. ) ;
#16210=VECTOR ( 'NONE', #13836, 1000.000000000000000 ) ;
#16229=CARTESIAN_POINT ( 'NONE',  ( -4.163336342344337027E-14, 1.387778780781445676E-14, 62.49999999999999289 ) ) ;
#16234=CARTESIAN_POINT ( 'NONE',  ( -35.78336344873367381, 4.414649291699865863, 34.71346399078494471 ) ) ;
#16246=CARTESIAN_POINT ( 'NONE',  ( 23.21352257770656990, 10.78826658734920230, -16.55003854064094426 ) ) ;
#16252=CARTESIAN_POINT ( 'NONE',  ( -29.81954908927651360, 15.48017614753370985, 41.40177460054280800 ) ) ;
#16267=CARTESIAN_POINT ( 'NONE',  ( 19.49999999999992539, 1.387778780781445676E-14, 51.25735931288069480 ) ) ;
#16271=CARTESIAN_POINT ( 'NONE',  ( 28.82515617888658355, -28.76482263229141978, 34.54546745300068977 ) ) ;
#16287=ADVANCED_FACE ( 'NONE', ( #4265 ), #4724, .F. ) ;
#16294=ORIENTED_EDGE ( 'NONE', *, *, #4808, .T. ) ;
#16322=ORIENTED_EDGE ( 'NONE', *, *, #13499, .T. ) ;
#16327=CARTESIAN_POINT ( 'NONE',  ( -29.92052531042452301, 27.29380315016930325, 30.33179664086772576 ) ) ;
#16331=CARTESIAN_POINT ( 'NONE',  ( -24.35970437652574105, -13.37404834226503070, 47.21042702067970254 ) ) ;
#16349=CARTESIAN_POINT ( 'NONE',  ( 9.268856789657291984, 38.25380398711768493, 34.80090346875810070 ) ) ;
#16386=CARTESIAN_POINT ( 'NONE',  ( -24.41454739814620822, 29.13939308268315287, 27.50000000000000711 ) ) ;
#16400=CARTESIAN_POINT ( 'NONE',  ( 27.66896717189014510, 25.39816801983182515, 27.50000000000000355 ) ) ;
#16407=CARTESIAN_POINT ( 'NONE',  ( -32.28307784207223108, 8.475829241206282560, -16.55003854064094426 ) ) ;
#16413=EDGE_CURVE ( 'NONE', #13876, #27501, #27594, .T. ) ;
#16416=ORIENTED_EDGE ( 'NONE', *, *, #4806, .T. ) ;
#16427=CARTESIAN_POINT ( 'NONE',  ( 23.42821736844243929, -34.00757704900313172, 29.63783715387382856 ) ) ;
#16431=DIRECTION ( 'NONE',  ( -0.3598999890241668664, 0.9329908884337534403, 0.000000000000000000 ) ) ;
#16478=CARTESIAN_POINT ( 'NONE',  ( -29.47411470116815835, 23.31420789013893824, 37.50000000004725109 ) ) ;
#16488=CARTESIAN_POINT ( 'NONE',  ( 26.58597676761595352, -6.321098805557485711, 43.43030304422416066 ) ) ;
#16491=CARTESIAN_POINT ( 'NONE',  ( 26.81381729043377860, -6.366069288663353198, 47.44085139292776887 ) ) ;
#16494=DIRECTION ( 'NONE',  ( 0.7071067811865487940, 0.000000000000000000, -0.7071067811865463515 ) ) ;
#16501=EDGE_CURVE ( 'NONE', #23899, #10056, #3058, .T. ) ;
#16510=ORIENTED_EDGE ( 'NONE', *, *, #24351, .F. ) ;
#16524=CARTESIAN_POINT ( 'NONE',  ( 18.22691194910808576, -34.07746802688367893, 34.49999999999999289 ) ) ;
#16528=ORIENTED_EDGE ( 'NONE', *, *, #22090, .T. ) ;
#16543=EDGE_CURVE ( 'NONE', #13000, #3499, #14554, .T. ) ;
#16547=CARTESIAN_POINT ( 'NONE',  ( 30.94848640118418714, 20.21248784850468638, 27.49999999999999289 ) ) ;
#16571=CARTESIAN_POINT ( 'NONE',  ( 29.66037709627321917, 27.60437511129337196, 30.29918945543065334 ) ) ;
#16572=EDGE_CURVE ( 'NONE', #10874, #7455, #15699, .T. ) ;
#16580=B_SPLINE_CURVE_WITH_KNOTS ( 'NONE', 3,
 ( #10626, #19986, #790, #643, #17648, #2833, #5792, #24348, #29505, #5488, #8141, #21859 ),
 .UNSPECIFIED., .F., .F.,
 ( 4, 2, 2, 2, 2, 4 ),
 ( 2.975219550396606016E-07, 0.0009689891316535842632, 0.001937680741352128993, 0.002906372351050673722, 0.003390718155899950965, 0.003875063960749227775 ),
 .UNSPECIFIED. ) ;
#16582=VERTEX_POINT ( 'NONE', #29521 ) ;
#16603=CARTESIAN_POINT ( 'NONE',  ( -23.07950435457407679, -11.50806656539752737, 49.21048435262065368 ) ) ;
#16607=EDGE_CURVE ( 'NONE', #30448, #20257, #21265, .T. ) ;
#16632=CARTESIAN_POINT ( 'NONE',  ( -24.31965562422391969, 28.55126061725682973, 37.50000000003461764 ) ) ;
#16634=LINE ( 'NONE', #26138, #28296 ) ;
#16663=ORIENTED_EDGE ( 'NONE', *, *, #22907, .T. ) ;
#16667=ORIENTED_EDGE ( 'NONE', *, *, #5362, .T. ) ;
#16672=ADVANCED_FACE ( 'NONE', ( #28554 ), #11253, .F. ) ;
#16684=CARTESIAN_POINT ( 'NONE',  ( -31.56327786402390245, -10.34181101807378944, -16.55003854064094426 ) ) ;
#16701=EDGE_LOOP ( 'NONE', ( #16667, #11600, #22511, #22995 ) ) ;
#16706=CARTESIAN_POINT ( 'NONE',  ( 34.93512232095646652, 9.847170278758666129, 27.50000000000000711 ) ) ;
#16721=DIRECTION ( 'NONE',  ( 0.7071067811865487940, 0.000000000000000000, -0.7071067811865463515 ) ) ;
#16727=CARTESIAN_POINT ( 'NONE',  ( 38.30271738069522058, 8.424491356373369655, 35.00506926609056535 ) ) ;
#16755=CARTESIAN_POINT ( 'NONE',  ( -23.12946144662536341, 11.96621729904739695, 44.71596222159476497 ) ) ;
#16778=CARTESIAN_POINT ( 'NONE',  ( -35.72251933182172934, 17.10365394847838161, 31.35234673342428380 ) ) ;
#16786=EDGE_CURVE ( 'NONE', #7581, #8115, #26478, .T. ) ;
#16794=CARTESIAN_POINT ( 'NONE',  ( 0.000000000000000000, 42.50000000000000000, 27.50000000000000355 ) ) ;
#16801=FACE_OUTER_BOUND ( 'NONE', #5611, .T. ) ;
#16819=VECTOR ( 'NONE', #30248, 1000.000000000000000 ) ;
#16825=ORIENTED_EDGE ( 'NONE', *, *, #22130, .F. ) ;
#16830=CARTESIAN_POINT ( 'NONE',  ( 23.63178464412187907, 33.91383858794676343, 29.64624590982186447 ) ) ;
#16851=CARTESIAN_POINT ( 'NONE',  ( -34.32465979325662886, 12.16814152140377558, 27.50000000000000355 ) ) ;
#16873=CARTESIAN_POINT ( 'NONE',  ( 33.51937758206383222, -10.82799271170304323, 39.77598051165973914 ) ) ;
#16883=LINE ( 'NONE', #338, #24745 ) ;
#16887=VECTOR ( 'NONE', #9454, 1000.000000000000000 ) ;
#16890=CARTESIAN_POINT ( 'NONE',  ( 24.38609055551176397, 33.28642614059371141, 34.50551068831410362 ) ) ;
#16896=EDGE_LOOP ( 'NONE', ( #7617, #14094, #30480, #15319 ) ) ;
#16914=CARTESIAN_POINT ( 'NONE',  ( -4.163336342344337027E-14, 1.387778780781445676E-14, 37.50000000000000000 ) ) ;
#16915=B_SPLINE_CURVE_WITH_KNOTS ( 'NONE', 3,
 ( #5089, #23950, #23794, #2753 ),
 .UNSPECIFIED., .F., .F.,
 ( 4, 4 ),
 ( 3.018024802580205417E-07, 0.007932103453629119755 ),
 .UNSPECIFIED. ) ;
#16936=DIRECTION ( 'NONE',  ( 0.9329908884337539954, -0.3598999890241654231, 0.000000000000000000 ) ) ;
#16939=CARTESIAN_POINT ( 'NONE',  ( -27.47456215299179050, 30.17515099587704341, 34.53186466379878539 ) ) ;
#16942=CARTESIAN_POINT ( 'NONE',  ( 33.56327786402390245, 10.22184702512350363, 35.67222522295137566 ) ) ;
#16952=CARTESIAN_POINT ( 'NONE',  ( -77.99999999999998579, -42.49999999999998579, 27.50000000000000000 ) ) ;
#16955=CARTESIAN_POINT ( 'NONE',  ( 2.338573377552017440, 39.50000000000000711, 27.50000000000001776 ) ) ;
#16970=ORIENTED_EDGE ( 'NONE', *, *, #26550, .T. ) ;
#16971=CARTESIAN_POINT ( 'NONE',  ( 24.35970437652574816, -13.37404834226503958, 42.96778633356033339 ) ) ;
#16974=EDGE_CURVE ( 'NONE', #5082, #17339, #20119, .T. ) ;
#16981=ORIENTED_EDGE ( 'NONE', *, *, #29590, .F. ) ;
#16983=CARTESIAN_POINT ( 'NONE',  ( 21.52288024096207764, -31.67788091438591991, 34.49999999999999289 ) ) ;
#16987=ORIENTED_EDGE ( 'NONE', *, *, #27313, .T. ) ;
#17022=AXIS2_PLACEMENT_3D ( 'NONE', #22021, #17190, #10027 ) ;
#17030=ADVANCED_FACE ( 'NONE', ( #4927 ), #2120, .F. ) ;
#17037=CARTESIAN_POINT ( 'NONE',  ( 32.80643058142531743, 23.14278286313888700, 34.65133582147071678 ) ) ;
#17044=VERTEX_POINT ( 'NONE', #7582 ) ;
#17045=ORIENTED_EDGE ( 'NONE', *, *, #27910, .T. ) ;
#17050=CARTESIAN_POINT ( 'NONE',  ( -23.08950671686661948, 11.27322061222802496, 49.30570747941608545 ) ) ;
#17059=ORIENTED_EDGE ( 'NONE', *, *, #30170, .T. ) ;
#17073=ORIENTED_EDGE ( 'NONE', *, *, #5594, .T. ) ;
#17081=DIRECTION ( 'NONE',  ( -0.000000000000000000, -0.000000000000000000, -1.000000000000000000 ) ) ;
#17083=VERTEX_POINT ( 'NONE', #15045 ) ;
#17087=CARTESIAN_POINT ( 'NONE',  ( -38.27812018866794830, -8.165225598437423571, 32.01105402497861263 ) ) ;
#17089=CARTESIAN_POINT ( 'NONE',  ( 23.21352257770656990, 10.78826658734920230, 45.15942333309104129 ) ) ;
#17105=VERTEX_POINT ( 'NONE', #24256 ) ;
#17132=CARTESIAN_POINT ( 'NONE',  ( -38.89958629580320348, 3.114405769308834948, 32.20030128012836457 ) ) ;
#17139=CARTESIAN_POINT ( 'NONE',  ( 23.83037915021597186, -29.68074934824784350, 34.49999999999999289 ) ) ;
#17142=ORIENTED_EDGE ( 'NONE', *, *, #21576, .F. ) ;
#17153=CARTESIAN_POINT ( 'NONE',  ( -23.84426482588630947, -29.66596207160800347, 34.49999999999999289 ) ) ;
#17154=CARTESIAN_POINT ( 'NONE',  ( -35.86437274510341666, 3.536632535693895019, 34.72985588596475992 ) ) ;
#17162=ORIENTED_EDGE ( 'NONE', *, *, #3316, .T. ) ;
#17166=LINE ( 'NONE', #24174, #631 ) ;
#17170=FACE_OUTER_BOUND ( 'NONE', #10456, .T. ) ;
#17189=CARTESIAN_POINT ( 'NONE',  ( 26.73499487113253892, 26.30340432104372894, 37.50000000004516210 ) ) ;
#17190=DIRECTION ( 'NONE',  ( -0.000000000000000000, -0.000000000000000000, 1.000000000000000000 ) ) ;
#17201=CARTESIAN_POINT ( 'NONE',  ( -32.28307784207223108, -8.475829241206275455, 41.62281023987519291 ) ) ;
#17203=CARTESIAN_POINT ( 'NONE',  ( -27.20149534458562712, 25.89115957524252210, 34.49999999999998579 ) ) ;
#17210=ADVANCED_FACE ( 'NONE', ( #23575 ), #26553, .F. ) ;
#17243=CARTESIAN_POINT ( 'NONE',  ( -37.89343041208743301, -10.07310561413692440, 31.90045860481988882 ) ) ;
#17283=CARTESIAN_POINT ( 'NONE',  ( 12.09996233686562128, 37.29787398801550324, 27.50000000000001066 ) ) ;
#17286=CARTESIAN_POINT ( 'NONE',  ( 38.79281043785276495, -5.073460407337612388, 32.16650784045132383 ) ) ;
#17291=CARTESIAN_POINT ( 'NONE',  ( -37.56589145670645280, -11.49135466129804684, 31.80857576914547380 ) ) ;
#17302=CARTESIAN_POINT ( 'NONE',  ( 32.60829997825918980, 13.18983524832148646, 35.60092001944725126 ) ) ;
#17323=DIRECTION ( 'NONE',  ( -0.000000000000000000, -0.000000000000000000, 1.000000000000000000 ) ) ;
#17329=CARTESIAN_POINT ( 'NONE',  ( 32.99222498713436380, 15.81026154464086986, 34.49999999999998579 ) ) ;
#17339=VERTEX_POINT ( 'NONE', #18924 ) ;
#17355=CARTESIAN_POINT ( 'NONE',  ( -23.36057818983818279, -12.54850586925978284, 44.23991181465311229 ) ) ;
#17392=CARTESIAN_POINT ( 'NONE',  ( -3.668093106282626081, -42.33811009507338952, 34.60879219164162635 ) ) ;
#17402=VERTEX_POINT ( 'NONE', #17817 ) ;
#17408=CARTESIAN_POINT ( 'NONE',  ( -24.41908749150431035, -33.17108856314850840, 34.50932754554303017 ) ) ;
#17418=CARTESIAN_POINT ( 'NONE',  ( 30.38302862529102200, 15.53680216053818874, 36.63232123326682199 ) ) ;
#17438=CARTESIAN_POINT ( 'NONE',  ( -27.98100949438103413, -24.85668482956322123, 27.50000000000001066 ) ) ;
#17446=ORIENTED_EDGE ( 'NONE', *, *, #4806, .F. ) ;
#17451=DIRECTION ( 'NONE',  ( -0.9895723101232632990, 0.1430086711943935607, 0.01718030851067640571 ) ) ;
#17455=CARTESIAN_POINT ( 'NONE',  ( -17.28117534813046774, 38.12494209667251255, 29.23509795125549005 ) ) ;
#17458=B_SPLINE_CURVE_WITH_KNOTS ( 'NONE', 3,
 ( #10146, #19651, #29172, #24492, #3136, #12659, #22153, #27007, #6656, #16173, #27730, #1984, #30512, #28028 ),
 .UNSPECIFIED., .F., .F.,
 ( 4, 2, 2, 2, 2, 2, 4 ),
 ( 2.108610145883729832E-07, 0.0004867403503157766501, 0.0009732698396169649517, 0.001459799328918153253, 0.001946328818219341663, 0.002919387796821711761, 0.003892446775424082510 ),
 .UNSPECIFIED. ) ;
#17488=CARTESIAN_POINT ( 'NONE',  ( 24.03448224033878944, 8.660042335149841009, 49.47829057475697567 ) ) ;
#17490=CARTESIAN_POINT ( 'NONE',  ( 25.91119823319791848, 27.43797854297901750, 34.50000000000000000 ) ) ;
#17492=CARTESIAN_POINT ( 'NONE',  ( -11.52197458429825083, 37.50933785548062360, 27.50000000000001066 ) ) ;
#17496=CARTESIAN_POINT ( 'NONE',  ( -24.58208797071834795, -7.298293523701643082, 49.35779847067230719 ) ) ;
#17499=CARTESIAN_POINT ( 'NONE',  ( 33.42925964089140933, 11.06161099612213405, 35.54550565580007060 ) ) ;
#17506=CARTESIAN_POINT ( 'NONE',  ( 0.000000000000000000, 42.50000000000000000, 27.50000000000000355 ) ) ;
#17507=CARTESIAN_POINT ( 'NONE',  ( 17.79450790306045604, 37.82695112826932160, 34.52540950801754605 ) ) ;
#17519=CARTESIAN_POINT ( 'NONE',  ( -19.49586959400445707, 33.20761599285713572, 34.49999999999998579 ) ) ;
#17532=DIRECTION ( 'NONE',  ( 0.1411672138529631859, 0.9899857664294936521, 0.000000000000000000 ) ) ;
#17538=CARTESIAN_POINT ( 'NONE',  ( -33.42925964089141644, -11.06161099612212695, 35.54550565580013455 ) ) ;
#17543=CARTESIAN_POINT ( 'NONE',  ( 0.4876298400482597661, -42.50362390527760681, 28.83943401234160930 ) ) ;
#17552=CIRCLE ( 'NONE', #27024, 22.49999999999996447 ) ;
#17554=CARTESIAN_POINT ( 'NONE',  ( -27.23683592356784544, -25.89410312378974410, 37.49999999984879651 ) ) ;
#17574=CARTESIAN_POINT ( 'NONE',  ( 33.21329855679435639, -9.207353758468070026, 40.53414655261587995 ) ) ;
#17582=CARTESIAN_POINT ( 'NONE',  ( -35.15416861624421330, -8.598791122201292936, 27.50000000000000355 ) ) ;
#17588=ORIENTED_EDGE ( 'NONE', *, *, #6123, .F. ) ;
#17593=ORIENTED_EDGE ( 'NONE', *, *, #6776, .T. ) ;
#17606=CARTESIAN_POINT ( 'NONE',  ( -4.506343322667617279, 42.22116422339769315, 28.86378313756725333 ) ) ;
#17633=EDGE_CURVE ( 'NONE', #9483, #15816, #25319, .T. ) ;
#17638=CARTESIAN_POINT ( 'NONE',  ( 31.46108752401734066, -15.19043599309334169, 35.82118098715091747 ) ) ;
#17643=CARTESIAN_POINT ( 'NONE',  ( 34.45950848030155100, 11.47319617667155711, 34.50000000000000000 ) ) ;
#17646=CARTESIAN_POINT ( 'NONE',  ( 30.38302862529101489, 15.53680216053818519, 40.87496192038609877 ) ) ;
#17648=CARTESIAN_POINT ( 'NONE',  ( 25.88640477275122009, 6.345529225273955909, 48.34755156421744005 ) ) ;
#17651=CARTESIAN_POINT ( 'NONE',  ( -23.09047454507859243, 11.74540567832115912, 44.85144129262233292 ) ) ;
#17652=ORIENTED_EDGE ( 'NONE', *, *, #16413, .F. ) ;
#17661=CARTESIAN_POINT ( 'NONE',  ( -33.03705654931147251, -8.970011997839668183, 36.52435908506018336 ) ) ;
#17667=B_SPLINE_CURVE_WITH_KNOTS ( 'NONE', 3,
 ( #12041, #4402, #16873, #14528 ),
 .UNSPECIFIED., .F., .F.,
 ( 4, 4 ),
 ( 0.002976194933398901288, 0.003711256114093793891 ),
 .UNSPECIFIED. ) ;
#17671=EDGE_CURVE ( 'NONE', #1048, #22947, #11180, .T. ) ;
#17677=PLANE ( 'NONE',  #138 ) ;
#17696=CARTESIAN_POINT ( 'NONE',  ( -23.07950435457407679, -11.50806656539752737, 44.96784366550136980 ) ) ;
#17701=CARTESIAN_POINT ( 'NONE',  ( -37.14285906899156231, -13.21667505289354061, 31.69282016062263807 ) ) ;
#17750=CARTESIAN_POINT ( 'NONE',  ( 11.97149782862661027, -40.45422486509310289, 29.01997631939856959 ) ) ;
#17757=CARTESIAN_POINT ( 'NONE',  ( -6.419316938171813369, 41.92620935963721962, 28.88939473975622718 ) ) ;
#17771=B_SPLINE_CURVE_WITH_KNOTS ( 'NONE', 3,
 ( #29574, #20053, #10228, #17418, #3532, #27230, #27547, #24572, #5555, #13049, #13356, #29892, #6173, #26937, #15676, #5705 ),
 .UNSPECIFIED., .F., .F.,
 ( 4, 2, 2, 2, 2, 2, 2, 4 ),
 ( 2.980374332640320740E-07, 0.0009280375596593695665, 0.001391907320772415311, 0.001855777081885461163, 0.002319646842998507232, 0.002783516604111560457, 0.003247386365224614116, 0.003711256126337667341 ),
 .UNSPECIFIED. ) ;
#17773=AXIS2_PLACEMENT_3D ( 'NONE', #3503, #22204, #17532 ) ;
#17787=ORIENTED_EDGE ( 'NONE', *, *, #10890, .F. ) ;
#17804=CARTESIAN_POINT ( 'NONE',  ( -17.94248964168179938, 34.33858135081683827, 27.49999999999999645 ) ) ;
#17814=VERTEX_POINT ( 'NONE', #4179 ) ;
#17817=CARTESIAN_POINT ( 'NONE',  ( 23.21352257770656990, 10.78826658734920230, 49.40206402021032517 ) ) ;
#17818=EDGE_CURVE ( 'NONE', #28109, #22736, #21471, .T. ) ;
#17824=CARTESIAN_POINT ( 'NONE',  ( 6.563702251502810725, 36.99658191090264125, 37.50000000022351543 ) ) ;
#17829=CARTESIAN_POINT ( 'NONE',  ( -33.37677408195396112, 9.488883682882484294, 40.30072466173501056 ) ) ;
#17857=CARTESIAN_POINT ( 'NONE',  ( -32.68301789103641397, 8.668739453992939659, 36.94438844897151597 ) ) ;
#17879=CARTESIAN_POINT ( 'NONE',  ( 32.14097302481091845, -14.40131566728160628, 39.78047203870804083 ) ) ;
#17892=ORIENTED_EDGE ( 'NONE', *, *, #9763, .F. ) ;
#17915=ORIENTED_EDGE ( 'NONE', *, *, #15859, .F. ) ;
#17919=CARTESIAN_POINT ( 'NONE',  ( 37.27204780043465604, -12.57768201427415988, 31.72981289407691108 ) ) ;
#17932=CARTESIAN_POINT ( 'NONE',  ( 27.03943647958860552, 26.20092231554394857, 27.49999999999999645 ) ) ;
#17933=EDGE_CURVE ( 'NONE', #526, #6797, #21630, .T. ) ;
#17943=CARTESIAN_POINT ( 'NONE',  ( 23.07601128794333434, 11.40611796340042261, 49.25937209212059997 ) ) ;
#17959=CARTESIAN_POINT ( 'NONE',  ( -17.94248964168179938, -34.33858135081683827, 34.80090346875805096 ) ) ;
#17963=VERTEX_POINT ( 'NONE', #2611 ) ;
#17967=VECTOR ( 'NONE', #25715, 1000.000000000000000 ) ;
#17982=ADVANCED_FACE ( 'NONE', ( #16801 ), #23964, .F. ) ;
#18006=EDGE_CURVE ( 'NONE', #22947, #18116, #19382, .T. ) ;
#18013=CARTESIAN_POINT ( 'NONE',  ( -33.25379661643704310, 9.265521131796548460, 36.23697955560132300 ) ) ;
#18025=CARTESIAN_POINT ( 'NONE',  ( -20.23374174526511027, -31.57860962931301785, 37.50000000001161027 ) ) ;
#18031=CARTESIAN_POINT ( 'NONE',  ( 33.56327786402390245, 10.34181101807379299, 35.63689980405264635 ) ) ;
#18038=DIRECTION ( 'NONE',  ( -0.000000000000000000, -0.000000000000000000, 1.000000000000000000 ) ) ;
#18041=CARTESIAN_POINT ( 'NONE',  ( 33.48316501811950019, -9.771059948263134842, 40.12037505765862733 ) ) ;
#18044=VERTEX_POINT ( 'NONE', #25199 ) ;
#18057=CARTESIAN_POINT ( 'NONE',  ( 4.216636297896264374, 37.26217892624189432, 37.50000000000000000 ) ) ;
#18058=ORIENTED_EDGE ( 'NONE', *, *, #28805, .F. ) ;
#18075=EDGE_LOOP ( 'NONE', ( #3366, #16102, #9719, #3018 ) ) ;
#18077=CARTESIAN_POINT ( 'NONE',  ( 21.86019681245147339, 31.48592878035296749, 34.80090346875810070 ) ) ;
#18078=ORIENTED_EDGE ( 'NONE', *, *, #20998, .T. ) ;
#18088=CARTESIAN_POINT ( 'NONE',  ( -27.86235613436986114, 14.72519157938688750, 43.48653168448687012 ) ) ;
#18089=CARTESIAN_POINT ( 'NONE',  ( 23.11610519334012537, 11.09643357455199464, 49.35895363836304028 ) ) ;
#18093=CARTESIAN_POINT ( 'NONE',  ( -33.52437897089259877, -10.76376600292166863, 39.79035104387400423 ) ) ;
#18107=CARTESIAN_POINT ( 'NONE',  ( -9.268856789657290207, -38.25380398711768493, 27.50000000000000355 ) ) ;
#18116=VERTEX_POINT ( 'NONE', #27408 ) ;
#18125=CARTESIAN_POINT ( 'NONE',  ( -10.33689618797787446, 37.84157881464940942, 27.50000000000000355 ) ) ;
#18127=CARTESIAN_POINT ( 'NONE',  ( -24.44496207165490276, -7.595930209050158588, -16.55003854064094426 ) ) ;
#18130=EDGE_CURVE ( 'NONE', #165, #28122, #24960, .T. ) ;
#18132=CARTESIAN_POINT ( 'NONE',  ( -32.28307784207223108, 8.475829241206282560, 41.62281023987520001 ) ) ;
#18141=EDGE_CURVE ( 'NONE', #3185, #7581, #30533, .T. ) ;
#18155=DIRECTION ( 'NONE',  ( -0.3598999890241659783, 0.9329908884337537733, 0.000000000000000000 ) ) ;
#18164=CARTESIAN_POINT ( 'NONE',  ( 35.03831055084558699, -13.42466405557608944, 37.50000000000372324 ) ) ;
#18175=CARTESIAN_POINT ( 'NONE',  ( -23.12263228470262888, -11.97179573940914921, 48.96234658225964864 ) ) ;
#18176=EDGE_CURVE ( 'NONE', #2982, #11117, #24691, .T. ) ;
#18208=CARTESIAN_POINT ( 'NONE',  ( -30.50204315964898427, -15.53056155674291183, 36.52918211141458471 ) ) ;
#18214=ORIENTED_EDGE ( 'NONE', *, *, #5526, .F. ) ;
#18229=CARTESIAN_POINT ( 'NONE',  ( -4.375757216953428294E-15, -39.50000000000000000, 27.50000000000000355 ) ) ;
#18235=CARTESIAN_POINT ( 'NONE',  ( 33.01877980957530667, -12.12572312222180670, 35.60092001944722995 ) ) ;
#18241=CARTESIAN_POINT ( 'NONE',  ( 31.56327786402390245, -10.34181101807379655, -16.55003854064094426 ) ) ;
#18242=EDGE_LOOP ( 'NONE', ( #21712, #6429, #6620, #1810 ) ) ;
#18259=CARTESIAN_POINT ( 'NONE',  ( -32.31576317091163730, 17.59561277345963504, 27.50000000000000355 ) ) ;
#18268=EDGE_LOOP ( 'NONE', ( #14697, #26018, #9704, #30787 ) ) ;
#18271=DIRECTION ( 'NONE',  ( -0.000000000000000000, -0.000000000000000000, 1.000000000000000000 ) ) ;
#18273=CARTESIAN_POINT ( 'NONE',  ( -32.28307784207223108, -8.475829241206275455, 41.62281023987519291 ) ) ;
#18277=CARTESIAN_POINT ( 'NONE',  ( -18.65094025732183525, 33.78913767902538012, 27.50000000000000355 ) ) ;
#18290=CARTESIAN_POINT ( 'NONE',  ( -30.53339558441486190, -7.800891647352838909, 39.24389099736757913 ) ) ;
#18315=CIRCLE ( 'NONE', #15284, 22.49999999999996447 ) ;
#18320=CARTESIAN_POINT ( 'NONE',  ( 36.92711665837346402, -13.73927826681822317, 34.88776314540329082 ) ) ;
#18343=CARTESIAN_POINT ( 'NONE',  ( 23.11610519334012537, 11.09643357455199464, 45.11631295124375640 ) ) ;
#18357=EDGE_LOOP ( 'NONE', ( #24723, #8083, #16528, #15126 ) ) ;
#18385=CARTESIAN_POINT ( 'NONE',  ( 26.12047388987419083, -6.311255530320352136, 43.88527982295130414 ) ) ;
#18402=CARTESIAN_POINT ( 'NONE',  ( 27.03943647958860197, -26.20092231554396633, 34.80090346875810070 ) ) ;
#18407=ORIENTED_EDGE ( 'NONE', *, *, #942, .T. ) ;
#18409=DIRECTION ( 'NONE',  ( -0.000000000000000000, -0.000000000000000000, 1.000000000000000000 ) ) ;
#18415=CARTESIAN_POINT ( 'NONE',  ( -32.28307784207223108, -8.475829241206275455, 41.62281023987519291 ) ) ;
#18416=VERTEX_POINT ( 'NONE', #14371 ) ;
#18429=CARTESIAN_POINT ( 'NONE',  ( -11.52197458429825261, -37.50933785548060229, 34.80090346875804386 ) ) ;
#18445=CARTESIAN_POINT ( 'NONE',  ( -4.915268975789784278, 39.22418258073496844, 27.50000000000000355 ) ) ;
#18453=ORIENTED_EDGE ( 'NONE', *, *, #16572, .T. ) ;
#18476=CARTESIAN_POINT ( 'NONE',  ( 38.89666010881209957, -3.348336038578077822, 32.19909834651174663 ) ) ;
#18484=CARTESIAN_POINT ( 'NONE',  ( -5.127072261997696501, -42.13114360820387105, 28.87158698979378713 ) ) ;
#18489=CARTESIAN_POINT ( 'NONE',  ( -23.21352257770656990, 10.78826658734919519, 45.15942333309111234 ) ) ;
#18494=DIRECTION ( 'NONE',  ( 1.000000000000000000, 0.000000000000000000, 0.000000000000000000 ) ) ;
#18499=CARTESIAN_POINT ( 'NONE',  ( -25.07950435457407323, 11.50806656539752737, -16.55003854064094426 ) ) ;
#18525=DIRECTION ( 'NONE',  ( 0.3598999890241700306, -0.9329908884337522190, 0.000000000000000000 ) ) ;
#18541=CARTESIAN_POINT ( 'NONE',  ( 34.83396020575241891, -10.30249279383517624, 27.50000000000001066 ) ) ;
#18550=ORIENTED_EDGE ( 'NONE', *, *, #3708, .F. ) ;
#18553=CARTESIAN_POINT ( 'NONE',  ( -33.56595177138117947, -10.45696648424866204, 39.84323675257729747 ) ) ;
#18583=CARTESIAN_POINT ( 'NONE',  ( -20.17405764020900705, 32.71829193411804937, 27.50000000000000000 ) ) ;
#18597=AXIS2_PLACEMENT_3D ( 'NONE', #25788, #28128, #1920 ) ;
#18600=CARTESIAN_POINT ( 'NONE',  ( 4.948301831468912226, -39.21750186235175306, 27.50000000000001066 ) ) ;
#18620=CARTESIAN_POINT ( 'NONE',  ( 12.13427030824643715, -40.39764110210223436, 29.02507812129452347 ) ) ;
#18639=CARTESIAN_POINT ( 'NONE',  ( 23.94376008874366235, 13.17067969463889732, 43.43030304407326270 ) ) ;
#18642=CARTESIAN_POINT ( 'NONE',  ( 33.42925964089141644, -11.06161099612213228, 35.54550565580004928 ) ) ;
#18649=CARTESIAN_POINT ( 'NONE',  ( -24.35970437652574105, 13.37404834226503247, 42.96778633356043287 ) ) ;
#18665=CARTESIAN_POINT ( 'NONE',  ( -35.06085151626346175, 18.66574915858497619, 34.76280655890868587 ) ) ;
#18673=CARTESIAN_POINT ( 'NONE',  ( 24.57973596967191554, -7.302173446879564267, 45.11631295118271368 ) ) ;
#18682=DIRECTION ( 'NONE',  ( -0.000000000000000000, -0.000000000000000000, 1.000000000000000000 ) ) ;
#18690=FACE_OUTER_BOUND ( 'NONE', #19131, .T. ) ;
#18728=CARTESIAN_POINT ( 'NONE',  ( -29.73688679209877606, 22.29461321502727600, 27.50000000000000355 ) ) ;
#18743=CARTESIAN_POINT ( 'NONE',  ( 28.71210443682918978, -23.83196592705972705, 27.50000000000000000 ) ) ;
#18772=CARTESIAN_POINT ( 'NONE',  ( 17.79366536559482626, -37.84673028964422059, 29.26143670286390019 ) ) ;
#18778=VERTEX_POINT ( 'NONE', #1949 ) ;
#18793=DIRECTION ( 'NONE',  ( -0.000000000000000000, -0.000000000000000000, 1.000000000000000000 ) ) ;
#18794=DIRECTION ( 'NONE',  ( 0.000000000000000000, 0.000000000000000000, 1.000000000000000000 ) ) ;
#18797=VECTOR ( 'NONE', #9234, 1000.000000000000000 ) ;
#18819=VERTEX_POINT ( 'NONE', #25658 ) ;
#18825=CARTESIAN_POINT ( 'NONE',  ( -18.45311310706550856, 32.73271211070382236, 37.49999999995343103 ) ) ;
#18830=VECTOR ( 'NONE', #9921, 1000.000000000000000 ) ;
#18831=VERTEX_POINT ( 'NONE', #22682 ) ;
#18835=CARTESIAN_POINT ( 'NONE',  ( 25.07174449839132890, -6.739288358966160963, 44.79593483594005221 ) ) ;
#18846=CARTESIAN_POINT ( 'NONE',  ( 0.000000000000000000, 39.50000000000000000, 34.80090346875809360 ) ) ;
#18855=CARTESIAN_POINT ( 'NONE',  ( -32.28307784207223108, 8.475829241206282560, 41.62281023987520001 ) ) ;
#18862=ORIENTED_EDGE ( 'NONE', *, *, #2938, .T. ) ;
#18867=DIRECTION ( 'NONE',  ( 1.000000000000000000, 0.000000000000000000, 0.000000000000000000 ) ) ;
#18872=CARTESIAN_POINT ( 'NONE',  ( -23.26375789455195431, 12.37328455203049593, 48.65081625091716688 ) ) ;
#18874=ORIENTED_EDGE ( 'NONE', *, *, #25932, .F. ) ;
#18876=PLANE ( 'NONE',  #22209 ) ;
#18890=CARTESIAN_POINT ( 'NONE',  ( -33.27395842691333172, 15.08718781055274860, 27.50000000000000355 ) ) ;
#18891=EDGE_CURVE ( 'NONE', #14452, #29313, #28540, .T. ) ;
#18901=CARTESIAN_POINT ( 'NONE',  ( -1.722266914199011234, -42.46879315525252707, 28.84242400037395626 ) ) ;
#18905=CARTESIAN_POINT ( 'NONE',  ( 23.04694076046884987, -30.34744638473161160, 27.50000000000000355 ) ) ;
#18924=CARTESIAN_POINT ( 'NONE',  ( 22.49999999999992184, 1.387778780781445676E-14, 52.50000000000000000 ) ) ;
#18928=PLANE ( 'NONE',  #18597 ) ;
#18933=CARTESIAN_POINT ( 'NONE',  ( 39.00152643798587349, 0.5466461374812251472, 35.07981065047974312 ) ) ;
#18939=ORIENTED_EDGE ( 'NONE', *, *, #27178, .T. ) ;
#18944=EDGE_LOOP ( 'NONE', ( #25184, #1778, #16663, #21745 ) ) ;
#18965=CARTESIAN_POINT ( 'NONE',  ( 33.26787633654602416, -9.290711110048579968, 36.21660691973271895 ) ) ;
#18980=CARTESIAN_POINT ( 'NONE',  ( -23.47668842614531215, 34.05319493990059954, 29.63203809737341743 ) ) ;
#18982=CARTESIAN_POINT ( 'NONE',  ( 24.44496207165490276, 7.595930209050162141, 45.15942333309104129 ) ) ;
#18986=CARTESIAN_POINT ( 'NONE',  ( -4.163336342344337027E-14, 1.387778780781445676E-14, 62.49999999999999289 ) ) ;
#19006=VERTEX_POINT ( 'NONE', #6122 ) ;
#19016=VECTOR ( 'NONE', #30521, 1000.000000000000000 ) ;
#19022=CARTESIAN_POINT ( 'NONE',  ( -15.00088867516242175, -39.32768935608851990, 29.12215979044223246 ) ) ;
#19036=CARTESIAN_POINT ( 'NONE',  ( -32.57644024395770543, 16.81967142788571579, 27.50000000000000000 ) ) ;
#19039=CARTESIAN_POINT ( 'NONE',  ( -19.53847887038948272, -33.17743341422470849, 34.50000000000000711 ) ) ;
#19045=CARTESIAN_POINT ( 'NONE',  ( -5.127072262013854242, -42.13114360820154047, 28.87158698979397897 ) ) ;
#19048=CARTESIAN_POINT ( 'NONE',  ( 32.55221183676798091, 16.87602028573894231, 27.50000000000000711 ) ) ;
#19069=CARTESIAN_POINT ( 'NONE',  ( 38.93844114562506320, 2.472344433271586706, 32.21256721326712835 ) ) ;
#19080=ORIENTED_EDGE ( 'NONE', *, *, #13004, .T. ) ;
#19083=EDGE_LOOP ( 'NONE', ( #29206, #7880, #3046, #646, #4386, #21835, #17652, #2022, #29167 ) ) ;
#19085=CARTESIAN_POINT ( 'NONE',  ( -24.44496207165490276, -7.595930209050158588, 45.15942333309111234 ) ) ;
#19093=EDGE_CURVE ( 'NONE', #3168, #26303, #3634, .T. ) ;
#19099=AXIS2_PLACEMENT_3D ( 'NONE', #13743, #4375, #21365 ) ;
#19101=CARTESIAN_POINT ( 'NONE',  ( -19.50000000000000711, 1.387778780781445676E-14, 62.49999999999999289 ) ) ;
#19125=CARTESIAN_POINT ( 'NONE',  ( -36.22259173693688439, 9.790317618809798006, 37.49999999994849986 ) ) ;
#19131=EDGE_LOOP ( 'NONE', ( #21093, #19080, #6416, #1631 ) ) ;
#19154=DIRECTION ( 'NONE',  ( -0.000000000000000000, -0.000000000000000000, 1.000000000000000000 ) ) ;
#19196=CARTESIAN_POINT ( 'NONE',  ( 22.58682123248537366, -30.76127850100380101, 27.50000000000000711 ) ) ;
#19206=DIRECTION ( 'NONE',  ( -0.9329908884337522190, 0.3598999890241700306, 0.000000000000000000 ) ) ;
#19215=CARTESIAN_POINT ( 'NONE',  ( 38.89137791791456067, -3.432770781813833771, 35.06776335884041629 ) ) ;
#19220=VERTEX_POINT ( 'NONE', #8403 ) ;
#19221=CARTESIAN_POINT ( 'NONE',  ( 28.78283879316666827, -7.125616703334846314, 41.10667063058290438 ) ) ;
#19239=CARTESIAN_POINT ( 'NONE',  ( 27.86235613436985759, 14.72519157938689460, 43.48653168448679196 ) ) ;
#19268=EDGE_CURVE ( 'NONE', #254, #20928, #3240, .T. ) ;
#19274=CARTESIAN_POINT ( 'NONE',  ( -26.14179753137254636, 26.91385278145934024, 37.49999999999091216 ) ) ;
#19275=ORIENTED_EDGE ( 'NONE', *, *, #21160, .T. ) ;
#19313=VERTEX_POINT ( 'NONE', #23488 ) ;
#19329=VERTEX_POINT ( 'NONE', #16331 ) ;
#19334=FACE_OUTER_BOUND ( 'NONE', #27444, .T. ) ;
#19340=DIRECTION ( 'NONE',  ( 1.000000000000000000, 0.000000000000000000, 0.000000000000000000 ) ) ;
#19382=B_SPLINE_CURVE_WITH_KNOTS ( 'NONE', 3,
 ( #10866, #20208, #15684, #13367, #3381, #20374, #29900, #22404 ),
 .UNSPECIFIED., .F., .F.,
 ( 4, 2, 2, 4 ),
 ( 0.000000000000000000, 0.005288043134213118134, 0.007932064701319680236, 0.01057608626842624147 ),
 .UNSPECIFIED. ) ;
#19383=CARTESIAN_POINT ( 'NONE',  ( 34.13328053751565250, 15.58287797514595141, 37.50000000001482903 ) ) ;
#19399=CARTESIAN_POINT ( 'NONE',  ( -23.16735716920978660, 10.90794401664034474, 49.39349105325691625 ) ) ;
#19432=CARTESIAN_POINT ( 'NONE',  ( -38.80437957496877033, -4.450587475999619791, 35.05861520490779526 ) ) ;
#19470=ADVANCED_FACE ( 'NONE', ( #14746, #12269 ), #26301, .T. ) ;
#19473=CARTESIAN_POINT ( 'NONE',  ( 13.71656802822472088, 39.80869574967974245, 29.07849776505763018 ) ) ;
#19479=CARTESIAN_POINT ( 'NONE',  ( -7.055757556308441814, 41.80458111945913657, 28.90000488980968640 ) ) ;
#19481=CARTESIAN_POINT ( 'NONE',  ( -26.11179934312166040, -14.04991663536888780, 41.10667063058298254 ) ) ;
#19499=CARTESIAN_POINT ( 'NONE',  ( -34.17152791855434657, -12.46745445544742381, 34.49999999999998579 ) ) ;
#19502=CARTESIAN_POINT ( 'NONE',  ( 26.31094384852241319, 8.315730187098496984, -16.55003854064094426 ) ) ;
#19516=CARTESIAN_POINT ( 'NONE',  ( 4.079864335184373303, 39.26151969706030798, 34.49999999999998579 ) ) ;
#19534=CARTESIAN_POINT ( 'NONE',  ( 29.78800378361061263, 27.44470329932194019, 34.56933849413994864 ) ) ;
#19549=CARTESIAN_POINT ( 'NONE',  ( -31.11230703446257451, 19.97580969618028846, 34.49999999999998579 ) ) ;
#19550=DIRECTION ( 'NONE',  ( -0.000000000000000000, -0.000000000000000000, 1.000000000000000000 ) ) ;
#19582=CARTESIAN_POINT ( 'NONE',  ( -38.70399152336479176, 5.266273049938332562, 32.13928303338958159 ) ) ;
#19601=CARTESIAN_POINT ( 'NONE',  ( 29.61203839202725518, -15.40012917324033381, 37.38016955275580244 ) ) ;
#19602=VERTEX_POINT ( 'NONE', #18031 ) ;
#19616=CARTESIAN_POINT ( 'NONE',  ( 23.94669763007064134, -13.17250946182262972, 43.42684587397059204 ) ) ;
#19618=VECTOR ( 'NONE', #5299, 1000.000000000000000 ) ;
#19623=CARTESIAN_POINT ( 'NONE',  ( -33.91683774368993198, -20.99019730004604156, 30.97961946053406734 ) ) ;
#19633=ADVANCED_FACE ( 'NONE', ( #22232 ), #12896, .F. ) ;
#19641=CARTESIAN_POINT ( 'NONE',  ( -19.12102597850193675, -33.46912219541083999, 34.50000000000000000 ) ) ;
#19651=CARTESIAN_POINT ( 'NONE',  ( -24.50429677314016175, 7.442113211156452302, 45.14840481399660632 ) ) ;
#19658=CARTESIAN_POINT ( 'NONE',  ( -9.268856789657274220, 38.25380398711767072, 34.80090346875804386 ) ) ;
#19663=EDGE_CURVE ( 'NONE', #27284, #11315, #2470, .T. ) ;
#19678=CARTESIAN_POINT ( 'NONE',  ( 19.71846758372799613, 31.98570203240115717, 37.49999999996673949 ) ) ;
#19684=CARTESIAN_POINT ( 'NONE',  ( -24.35970437652574105, -13.37404834226503070, 42.96778633356041865 ) ) ;
#19685=SHAPE_REPRESENTATION ( 'Vane Snap Cap', ( #7396 ), #15375 ) ;
#19706=B_SPLINE_CURVE_WITH_KNOTS ( 'NONE', 3,
 ( #3508, #25327, #17857, #27375, #5995, #3655, #18013, #27522, #6143, #15649, #25161, #13330, #7210, #4255, #28584, #28434 ),
 .UNSPECIFIED., .F., .F.,
 ( 4, 2, 2, 2, 2, 2, 2, 4 ),
 ( 2.980251112119010967E-07, 0.0009280375473568674505, 0.001391907308479688144, 0.001855777069602508947, 0.002319646830725329966, 0.002783516591848150552, 0.003247386352970971137, 0.003711256114093792156 ),
 .UNSPECIFIED. ) ;
#19716=VERTEX_POINT ( 'NONE', #6767 ) ;
#19719=CARTESIAN_POINT ( 'NONE',  ( 0.4053375914187597462, -37.50239422248243670, 37.50000000001958256 ) ) ;
#19730=CARTESIAN_POINT ( 'NONE',  ( -34.63718683596842141, -19.58198806418189264, 34.73973886756552076 ) ) ;
#19731=ORIENTED_EDGE ( 'NONE', *, *, #16501, .T. ) ;
#19754=CYLINDRICAL_SURFACE ( 'NONE', #23594, 2.000000000000005329 ) ;
#19759=CARTESIAN_POINT ( 'NONE',  ( -32.62510195252448852, -16.87942069704176618, 27.50000000000000711 ) ) ;
#19764=CIRCLE ( 'NONE', #17773, 10.00000000000000000 ) ;
#19769=CARTESIAN_POINT ( 'NONE',  ( 0.6177220288906448697, 39.50000000000000711, 27.50000000000001066 ) ) ;
#19777=CARTESIAN_POINT ( 'NONE',  ( -23.21352257770656990, -10.78826658734919519, 49.40206402021038201 ) ) ;
#19778=CARTESIAN_POINT ( 'NONE',  ( -32.73678307250399655, 23.13608884642247787, 30.76341402026043070 ) ) ;
#19825=CARTESIAN_POINT ( 'NONE',  ( -9.268856789657274220, 38.25380398711767072, 27.50000000000000355 ) ) ;
#19828=VERTEX_POINT ( 'NONE', #27993 ) ;
#19829=CARTESIAN_POINT ( 'NONE',  ( -24.86084284002701494, -6.930828199065639517, 49.19141369485819126 ) ) ;
#19846=CARTESIAN_POINT ( 'NONE',  ( 27.03074382657074537, 6.449748410230989215, 42.96778633356034760 ) ) ;
#19855=EDGE_LOOP ( 'NONE', ( #22591, #11648, #23517, #132 ) ) ;
#19858=CARTESIAN_POINT ( 'NONE',  ( -21.52174834036059181, 31.67861116925338294, 34.49999999999998579 ) ) ;
#19882=CARTESIAN_POINT ( 'NONE',  ( 33.48316501811951440, -9.771059948263138395, 35.87773437053935055 ) ) ;
#19901=CARTESIAN_POINT ( 'NONE',  ( -29.21234432035051753, -23.52169588460707672, 37.50000000003778666 ) ) ;
#19902=VERTEX_POINT ( 'NONE', #2564 ) ;
#19946=VECTOR ( 'NONE', #21870, 1000.000000000000000 ) ;
#19948=CARTESIAN_POINT ( 'NONE',  ( -2.584357522460066559, 42.42979574273064713, 28.84576176055872665 ) ) ;
#19977=AXIS2_PLACEMENT_3D ( 'NONE', #10188, #19550, #12854 ) ;
#19978=CARTESIAN_POINT ( 'NONE',  ( 23.21352257770656990, 10.78826658734920230, 49.40206402021032517 ) ) ;
#19982=CARTESIAN_POINT ( 'NONE',  ( -21.86019681245148405, 31.48592878035298170, 27.50000000000001776 ) ) ;
#19984=CARTESIAN_POINT ( 'NONE',  ( 31.22486525274645430, 15.32888848509420043, 40.21560466201665918 ) ) ;
#19986=CARTESIAN_POINT ( 'NONE',  ( 26.81368379037234817, 6.366017791192971842, 47.44099319977354412 ) ) ;
#19997=CARTESIAN_POINT ( 'NONE',  ( 8.838492628486433134, 36.51832121211318594, 37.49999999994788169 ) ) ;
#20000=CARTESIAN_POINT ( 'NONE',  ( -33.56830061431172396, -10.30497729095454851, 35.64318943580060761 ) ) ;
#20027=VERTEX_POINT ( 'NONE', #10189 ) ;
#20029=ORIENTED_EDGE ( 'NONE', *, *, #4404, .F. ) ;
#20030=CARTESIAN_POINT ( 'NONE',  ( -31.10500197267670330, 15.38309308716405077, 36.05646065676234002 ) ) ;
#20041=LINE ( 'NONE', #10847, #11842 ) ;
#20042=CARTESIAN_POINT ( 'NONE',  ( -32.41727157990033703, -18.89317060219217126, 37.49999999997574918 ) ) ;
#20053=CARTESIAN_POINT ( 'NONE',  ( 29.81956388892670873, 15.48018185647901923, 37.15911814917521383 ) ) ;
#20055=DIRECTION ( 'NONE',  ( -0.000000000000000000, -0.000000000000000000, 1.000000000000000000 ) ) ;
#20091=CIRCLE ( 'NONE', #26580, 19.49999999999996447 ) ;
#20099=CARTESIAN_POINT ( 'NONE',  ( -1.297549323414336042, 42.50000000000001421, 28.83974596215564290 ) ) ;
#20119=LINE ( 'NONE', #22602, #16210 ) ;
#20132=CARTESIAN_POINT ( 'NONE',  ( 33.51212652704789008, 9.877957833750135919, 40.06253926477352678 ) ) ;
#20150=CARTESIAN_POINT ( 'NONE',  ( 17.19472854822046060, 38.15486337162199248, 34.52907637737875746 ) ) ;
#20160=CARTESIAN_POINT ( 'NONE',  ( 32.28307784207223108, 8.475829241206289666, -16.55003854064094426 ) ) ;
#20168=CYLINDRICAL_SURFACE ( 'NONE', #14617, 1.999999999999998224 ) ;
#20177=CARTESIAN_POINT ( 'NONE',  ( -31.22647667302023677, 15.32805873036034328, 35.97188228574919577 ) ) ;
#20187=CARTESIAN_POINT ( 'NONE',  ( -12.57346322279386364, -40.23757549468835037, 29.03955556716994124 ) ) ;
#20208=CARTESIAN_POINT ( 'NONE',  ( 35.13802340819238168, -8.772855875097450351, 34.58409965093443361 ) ) ;
#20218=VERTEX_POINT ( 'NONE', #21852 ) ;
#20225=DIRECTION ( 'NONE',  ( 1.000000000000000000, 0.000000000000000000, 0.000000000000000000 ) ) ;
#20241=CARTESIAN_POINT ( 'NONE',  ( 30.60812557944273848, -26.34642019089854870, 30.43068197896959504 ) ) ;
#20256=CARTESIAN_POINT ( 'NONE',  ( 27.03943647958860552, 26.20092231554394857, 34.80090346875808649 ) ) ;
#20257=VERTEX_POINT ( 'NONE', #10008 ) ;
#20259=EDGE_CURVE ( 'NONE', #17044, #3185, #25540, .T. ) ;
#20281=CARTESIAN_POINT ( 'NONE',  ( 31.57687401261850724, -15.10620312102102680, 35.75338942089695848 ) ) ;
#20290=CARTESIAN_POINT ( 'NONE',  ( -31.18890335284659443, -19.89223002944918051, 27.50000000000000355 ) ) ;
#20309=LINE ( 'NONE', #27342, #6454 ) ;
#20323=EDGE_LOOP ( 'NONE', ( #1607, #7971, #27165, #4722, #21186, #15908, #18453, #20422, #2006 ) ) ;
#20324=CARTESIAN_POINT ( 'NONE',  ( 16.58889461517681951, -35.15515261640817357, 27.50000000000000711 ) ) ;
#20329=CARTESIAN_POINT ( 'NONE',  ( 32.28307784207223108, -8.475829241206289666, 37.38016955275583086 ) ) ;
#20347=EDGE_LOOP ( 'NONE', ( #25136, #17593, #23007, #365 ) ) ;
#20359=CARTESIAN_POINT ( 'NONE',  ( -8.896251305007044863, -36.43423536520429451, 37.50000000002009415 ) ) ;
#20364=ORIENTED_EDGE ( 'NONE', *, *, #13503, .F. ) ;
#20365=CARTESIAN_POINT ( 'NONE',  ( 24.35970437652574105, 13.37404834226503958, 42.96778633356035471 ) ) ;
#20374=CARTESIAN_POINT ( 'NONE',  ( 35.97269501643856415, -1.773469557554536502, 34.75180443448059719 ) ) ;
#20389=VERTEX_POINT ( 'NONE', #8395 ) ;
#20414=CARTESIAN_POINT ( 'NONE',  ( -4.375757216953428294E-15, -39.50000000000000000, 34.80090346875809360 ) ) ;
#20420=EDGE_CURVE ( 'NONE', #19716, #2236, #1839, .T. ) ;
#20422=ORIENTED_EDGE ( 'NONE', *, *, #22275, .T. ) ;
#20428=PLANE ( 'NONE',  #21707 ) ;
#20431=CARTESIAN_POINT ( 'NONE',  ( -33.37783937289808733, -9.491076832576640143, 40.29910134393502119 ) ) ;
#20443=ORIENTED_EDGE ( 'NONE', *, *, #17671, .T. ) ;
#20465=CARTESIAN_POINT ( 'NONE',  ( -33.54113041553378594, 10.01041480049199173, 39.99718304311860351 ) ) ;
#20466=CARTESIAN_POINT ( 'NONE',  ( 28.78283879316666471, 7.125616703334845425, 45.34931131770219537 ) ) ;
#20482=ORIENTED_EDGE ( 'NONE', *, *, #16543, .F. ) ;
#20486=DIRECTION ( 'NONE',  ( -0.9329908884337537733, -0.3598999890241659783, 0.000000000000000000 ) ) ;
#20494=CARTESIAN_POINT ( 'NONE',  ( 11.91580570916392290, -40.47530258207431331, 34.56547942634522030 ) ) ;
#20546=ORIENTED_EDGE ( 'NONE', *, *, #6521, .F. ) ;
#20547=CARTESIAN_POINT ( 'NONE',  ( 33.42925964089141644, -11.06161099612213228, 39.78814634291933316 ) ) ;
#20548=CARTESIAN_POINT ( 'NONE',  ( 26.47682648895289503, -31.23348282226190165, 29.92111261860823745 ) ) ;
#20556=CARTESIAN_POINT ( 'NONE',  ( 15.85884089648733131, 35.55173462727347555, 34.80090346875810070 ) ) ;
#20560=AXIS2_PLACEMENT_3D ( 'NONE', #26819, #17451, #5281 ) ;
#20570=CARTESIAN_POINT ( 'NONE',  ( -29.61203839202723032, 15.40012917324033204, -16.55003854064094426 ) ) ;
#20578=VECTOR ( 'NONE', #9066, 1000.000000000000000 ) ;
#20582=CARTESIAN_POINT ( 'NONE',  ( -4.375757216953428294E-15, -39.50000000000000000, 27.50000000000000355 ) ) ;
#20624=EDGE_CURVE ( 'NONE', #19902, #13000, #224, .T. ) ;
#20628=CARTESIAN_POINT ( 'NONE',  ( -32.14097302481091134, 14.40131566728161161, 39.78047203870814741 ) ) ;
#20642=CARTESIAN_POINT ( 'NONE',  ( 8.636617860055906704, -41.55279347581889482, 34.58763896935784032 ) ) ;
#20645=CARTESIAN_POINT ( 'NONE',  ( 26.11179934312166395, 14.04991663536889490, 41.10667063058291859 ) ) ;
#20652=CARTESIAN_POINT ( 'NONE',  ( -5.029589720568788280, -42.14523135962111411, 34.60377126736915443 ) ) ;
#20658=CARTESIAN_POINT ( 'NONE',  ( 30.03865005752671280, -15.52610542268209848, 41.18623755349090487 ) ) ;
#20662=CARTESIAN_POINT ( 'NONE',  ( -33.01877980957529957, -12.12572312222180315, 39.84356070656659909 ) ) ;
#20684=CARTESIAN_POINT ( 'NONE',  ( -7.404849586872397360, 36.78056030116736963, 37.49999999995792166 ) ) ;
#20686=CARTESIAN_POINT ( 'NONE',  ( -24.35970437652574105, 13.37404834226503247, -16.55003854064094426 ) ) ;
#20689=PLANE ( 'NONE',  #24491 ) ;
#20693=CARTESIAN_POINT ( 'NONE',  ( 25.18466322232232457, -6.657711795334226856, 44.70772167919919582 ) ) ;
#20695=DIRECTION ( 'NONE',  ( 1.000000000000000000, 0.000000000000000000, 0.000000000000000000 ) ) ;
#20703=CARTESIAN_POINT ( 'NONE',  ( 35.76481447503399380, 5.202797454133643917, 27.50000000000001066 ) ) ;
#20704=EDGE_LOOP ( 'NONE', ( #25722, #14111, #5657, #11041 ) ) ;
#20714=CARTESIAN_POINT ( 'NONE',  ( -32.28307784207223108, -8.475829241206282560, 37.38016955275590902 ) ) ;
#20728=CARTESIAN_POINT ( 'NONE',  ( -24.44496207165490276, 7.595930209050158588, 45.15942333309111945 ) ) ;
#20735=CARTESIAN_POINT ( 'NONE',  ( 33.56327786402390245, 10.34181101807379299, 35.63689980405264635 ) ) ;
#20754=ORIENTED_EDGE ( 'NONE', *, *, #1025, .T. ) ;
#20789=CARTESIAN_POINT ( 'NONE',  ( 38.51154267803796927, -7.181154427913921445, 32.07953739683074446 ) ) ;
#20801=CARTESIAN_POINT ( 'NONE',  ( -10.40135423173695273, -40.96791945951391511, 34.57567134912213191 ) ) ;
#20818=AXIS2_PLACEMENT_3D ( 'NONE', #20686, #6805, #25686 ) ;
#20844=CARTESIAN_POINT ( 'NONE',  ( -13.84835643114477577, 39.75824490312070481, 34.55175125678480441 ) ) ;
#20846=CARTESIAN_POINT ( 'NONE',  ( 26.11179934312167461, -14.04991663536889313, 45.34931131770218116 ) ) ;
#20853=CARTESIAN_POINT ( 'NONE',  ( 24.75800239156184546, -7.045788922043120017, 45.01673140503397974 ) ) ;
#20866=CARTESIAN_POINT ( 'NONE',  ( 34.13832859401787800, -12.80067323710190053, 34.80090346875810781 ) ) ;
#20887=VECTOR ( 'NONE', #13721, 1000.000000000000000 ) ;
#20888=CARTESIAN_POINT ( 'NONE',  ( -36.00000000000000000, -2.601438916704193360, 27.50000000000001066 ) ) ;
#20901=CARTESIAN_POINT ( 'NONE',  ( 32.28307784207223108, -8.475829241206289666, -16.55003854064094426 ) ) ;
#20914=EDGE_LOOP ( 'NONE', ( #23059, #21418, #13454, #20482 ) ) ;
#20918=CARTESIAN_POINT ( 'NONE',  ( -4.375757216953428294E-15, -39.50000000000000000, 27.50000000000000355 ) ) ;
#20928=VERTEX_POINT ( 'NONE', #3274 ) ;
#20933=ORIENTED_EDGE ( 'NONE', *, *, #1597, .F. ) ;
#20936=CARTESIAN_POINT ( 'NONE',  ( 7.360936444143488799, -36.84655860943143324, 37.49999999987780086 ) ) ;
#20945=CARTESIAN_POINT ( 'NONE',  ( -31.22486525274646851, -15.32888848509419510, 40.21560466201672313 ) ) ;
#20948=CARTESIAN_POINT ( 'NONE',  ( -23.62400240902268322, 9.724154461249517212, 45.23564988763775574 ) ) ;
#20950=CARTESIAN_POINT ( 'NONE',  ( 23.26155266345719141, 12.35118985415807025, 44.42018155111519917 ) ) ;
#20970=CARTESIAN_POINT ( 'NONE',  ( -22.50000000000000711, 1.387778780781445676E-14, 62.49999999999999289 ) ) ;
#20973=ORIENTED_EDGE ( 'NONE', *, *, #16786, .T. ) ;
#20985=CARTESIAN_POINT ( 'NONE',  ( -27.32656920039229220, 30.33072541150529844, 30.01477169192959238 ) ) ;
#20998=EDGE_CURVE ( 'NONE', #17105, #2982, #16056, .T. ) ;
#21014=DIRECTION ( 'NONE',  ( 1.000000000000000000, 0.000000000000000000, 0.000000000000000000 ) ) ;
#21019=VECTOR ( 'NONE', #26744, 1000.000000000000000 ) ;
#21021=CARTESIAN_POINT ( 'NONE',  ( -33.48610676296128474, -10.91424270342314529, 39.78047203871652471 ) ) ;
#21037=CARTESIAN_POINT ( 'NONE',  ( -24.18487066411278619, 13.30660647122584983, 47.39613942427950377 ) ) ;
#21041=CARTESIAN_POINT ( 'NONE',  ( 7.044370898287875882, -38.75167233872380734, 34.49999999999997868 ) ) ;
#21062=B_SPLINE_CURVE_WITH_KNOTS ( 'NONE', 3,
 ( #215, #7555, #19239, #11763 ),
 .UNSPECIFIED., .F., .F.,
 ( 4, 4 ),
 ( 3.018024802580205417E-07, 0.007932103453629116285 ),
 .UNSPECIFIED. ) ;
#21065=CARTESIAN_POINT ( 'NONE',  ( 17.09326798506966938, 34.76714281734690815, 27.50000000000000355 ) ) ;
#21068=LINE ( 'NONE', #16246, #5527 ) ;
#21087=CARTESIAN_POINT ( 'NONE',  ( 32.88898149417357075, -18.05935166304826822, 37.50000000004457945 ) ) ;
#21093=ORIENTED_EDGE ( 'NONE', *, *, #27873, .F. ) ;
#21095=CARTESIAN_POINT ( 'NONE',  ( -31.57476163834523675, -15.10795358447669301, 35.75454235600954433 ) ) ;
#21097=ORIENTED_EDGE ( 'NONE', *, *, #18141, .F. ) ;
#21117=CARTESIAN_POINT ( 'NONE',  ( 33.42925964089141644, -11.06161099612213228, 35.54550565580004928 ) ) ;
#21132=CARTESIAN_POINT ( 'NONE',  ( -20.48943103728710469, 31.49987920171448508, 37.49999999989595523 ) ) ;
#21133=ORIENTED_EDGE ( 'NONE', *, *, #25501, .T. ) ;
#21144=FACE_OUTER_BOUND ( 'NONE', #20704, .T. ) ;
#21145=CARTESIAN_POINT ( 'NONE',  ( 25.88604317058895532, -6.345278376181630264, 48.34797144667699342 ) ) ;
#21160=EDGE_CURVE ( 'NONE', #23060, #9483, #13226, .T. ) ;
#21164=CARTESIAN_POINT ( 'NONE',  ( -25.07174449839133601, 6.739288358966155634, 49.03857552305944267 ) ) ;
#21168=B_SPLINE_CURVE_WITH_KNOTS ( 'NONE', 3,
 ( #954, #17488, #21850, #19978 ),
 .UNSPECIFIED., .F., .F.,
 ( 4, 4 ),
 ( 2.143643656977390230E-07, 0.003421830178490238052 ),
 .UNSPECIFIED. ) ;
#21174=DIRECTION ( 'NONE',  ( 0.000000000000000000, 0.000000000000000000, 1.000000000000000000 ) ) ;
#21185=DIRECTION ( 'NONE',  ( 1.000000000000000000, 0.000000000000000000, 0.000000000000000000 ) ) ;
#21186=ORIENTED_EDGE ( 'NONE', *, *, #24407, .T. ) ;
#21192=CARTESIAN_POINT ( 'NONE',  ( -23.16735716920977950, 10.90794401664034652, 45.15085036613763236 ) ) ;
#21193=( GEOMETRIC_REPRESENTATION_CONTEXT ( 3 ) GLOBAL_UNCERTAINTY_ASSIGNED_CONTEXT ( ( #2353 ) ) GLOBAL_UNIT_ASSIGNED_CONTEXT ( ( #10820, #10508, #22198 ) ) REPRESENTATION_CONTEXT ( 'NONE', 'WORKASPACE' ) );
#21199=DIRECTION ( 'NONE',  ( -1.000000000000000000, 0.000000000000000000, 0.000000000000000000 ) ) ;
#21211=CARTESIAN_POINT ( 'NONE',  ( 36.00220402031282418, -2.441524372556627132, 27.50000000000000355 ) ) ;
#21238=CARTESIAN_POINT ( 'NONE',  ( 39.00145586610816650, 0.5332248899570756207, 32.23263252817133662 ) ) ;
#21239=DIRECTION ( 'NONE',  ( -1.000000000000000000, 0.000000000000000000, 0.000000000000000000 ) ) ;
#21251=B_SPLINE_CURVE_WITH_KNOTS ( 'NONE', 3,
 ( #11706, #23400, #18445, #25455, #27947, #30572, #18125, #11415, #16086, #9212, #23236, #23543, #18277, #6573, #18583, #27639, #16386, #4531, #25606, #15774, #4222, #28091, #18728, #6717, #28239, #6868, #19036, #28550, #18890, #16851, #2337, #3390, #27101, #9368, #26957, #3230, #7342, #29444, #23861, #17582, #12752, #2504, #12603, #12019, #5580, #19759, #14506, #21367, #26366, #17438, #29288, #15074, #28401, #3084, #7181, #24590, #14348, #26202, #5, #4833, #5722, #24442, #4995, #22256, #22096, #15216, #11868, #14186, #727, #22413 ),
 .UNSPECIFIED., .F., .F.,
 ( 4, 2, 2, 2, 2, 2, 2, 2, 2, 2, 2, 2, 2, 2, 2, 2, 2, 2, 2, 2, 2, 2, 2, 2, 2, 2, 2, 2, 2, 2, 2, 2, 2, 2, 4 ),
 ( 0.1181738554856288231, 0.1255522872445846982, 0.1273968951843236774, 0.1292415031240626566, 0.1329307190035405872, 0.1366199348830185178, 0.1384645428227574970, 0.1403091507624964485, 0.1476875825214522819, 0.1495321904611912334, 0.1513767984009302126, 0.1550660142804081154, 0.1587552301598860460, 0.1605998380996250252, 0.1624444460393639766, 0.1698228777983198101, 0.1735120936777977130, 0.1753567016175366922, 0.1772013095572756436, 0.1845797413162314771, 0.1882689571957093799, 0.1901135651354483314, 0.1919581730751873105, 0.1993366048341431163, 0.2030258207136210746, 0.2048704286533600261, 0.2067150365930989775, 0.2140934683520547832, 0.2159380762917937346, 0.2177826842315326861, 0.2214719001110106167, 0.2288503318699664502, 0.2306949398097054016, 0.2325395477494443530, 0.2362287636289222559 ),
 .UNSPECIFIED. ) ;
#21265=B_SPLINE_CURVE_WITH_KNOTS ( 'NONE', 3,
 ( #3625, #13146, #27805, #6110 ),
 .UNSPECIFIED., .F., .F.,
 ( 4, 4 ),
 ( 2.143643656964904170E-07, 0.003421830178490233715 ),
 .UNSPECIFIED. ) ;
#21275=CARTESIAN_POINT ( 'NONE',  ( 33.21329855679436349, -9.207353758468071803, 36.29150586549661028 ) ) ;
#21298=CARTESIAN_POINT ( 'NONE',  ( -33.48680455852475291, 16.92615973923613737, 37.49999999998726707 ) ) ;
#21311=LINE ( 'NONE', #4637, #19016 ) ;
#21331=B_SPLINE_CURVE_WITH_KNOTS ( 'NONE', 3,
 ( #26118, #4144, #4749, #16152, #14103 ),
 .UNSPECIFIED., .F., .F.,
 ( 4, 1, 4 ),
 ( 6.145237473689745305E-19, 0.002536462521843869077, 0.005072925043687738153 ),
 .UNSPECIFIED. ) ;
#21353=CARTESIAN_POINT ( 'NONE',  ( 20.71901075410115922, -32.31713536268975417, 34.50000000000000000 ) ) ;
#21362=PLANE ( 'NONE',  #26291 ) ;
#21365=DIRECTION ( 'NONE',  ( 1.000000000000000000, 0.000000000000000000, 0.000000000000000000 ) ) ;
#21367=CARTESIAN_POINT ( 'NONE',  ( -29.73518274310997356, -22.29727607186046967, 27.50000000000001421 ) ) ;
#21374=CARTESIAN_POINT ( 'NONE',  ( -4.163336342344337027E-14, 1.387778780781445676E-14, 62.49999999999999289 ) ) ;
#21377=ADVANCED_FACE ( 'NONE', ( #1982 ), #28172, .F. ) ;
#21382=CARTESIAN_POINT ( 'NONE',  ( 35.93079460107085055, 2.525230334074545890, 27.50000000000000355 ) ) ;
#21405=CARTESIAN_POINT ( 'NONE',  ( 37.36706805913578222, 12.24402983531209621, 34.92319840363951045 ) ) ;
#21418=ORIENTED_EDGE ( 'NONE', *, *, #5741, .T. ) ;
#21422=EDGE_CURVE ( 'NONE', #11315, #4164, #27755, .T. ) ;
#21440=ORIENTED_EDGE ( 'NONE', *, *, #21422, .F. ) ;
#21446=ORIENTED_EDGE ( 'NONE', *, *, #18130, .T. ) ;
#21454=CARTESIAN_POINT ( 'NONE',  ( -36.92102040520508410, 13.75791949449672380, 34.88729987039940994 ) ) ;
#21466=DIRECTION ( 'NONE',  ( 1.000000000000000000, 0.000000000000000000, 0.000000000000000000 ) ) ;
#21470=ORIENTED_EDGE ( 'NONE', *, *, #14349, .F. ) ;
#21471=LINE ( 'NONE', #28362, #10263 ) ;
#21480=LINE ( 'NONE', #9488, #13679 ) ;
#21492=CARTESIAN_POINT ( 'NONE',  ( 27.03074382657074537, 6.449748410230989215, 42.96778633356034760 ) ) ;
#21497=CARTESIAN_POINT ( 'NONE',  ( -23.07950435457351190, 11.50806656539842798, 49.21048435262080289 ) ) ;
#21527=CARTESIAN_POINT ( 'NONE',  ( 35.98550141493651466, 1.281847341532557083, 27.50000000000000355 ) ) ;
#21536=CARTESIAN_POINT ( 'NONE',  ( -31.46108752401733000, 15.19043599309334525, 40.06382167427029373 ) ) ;
#21544=EDGE_CURVE ( 'NONE', #19329, #1203, #16915, .T. ) ;
#21552=CARTESIAN_POINT ( 'NONE',  ( 37.36871377735028688, -3.393397791468933278, 37.50000000003174705 ) ) ;
#21553=DIRECTION ( 'NONE',  ( -0.000000000000000000, -0.000000000000000000, -1.000000000000000000 ) ) ;
#21557=EDGE_LOOP ( 'NONE', ( #27479, #2638, #16970, #2874 ) ) ;
#21567=EDGE_LOOP ( 'NONE', ( #177, #16987, #17162, #2341 ) ) ;
#21576=EDGE_CURVE ( 'NONE', #19220, #14452, #5039, .T. ) ;
#21587=LINE ( 'NONE', #19101, #22238 ) ;
#21603=EDGE_CURVE ( 'NONE', #4914, #7455, #4624, .T. ) ;
#21612=CARTESIAN_POINT ( 'NONE',  ( -38.41462058491280374, 7.368026156770138613, 35.01883456753041912 ) ) ;
#21630=LINE ( 'NONE', #3223, #29693 ) ;
#21635=EDGE_CURVE ( 'NONE', #11117, #22736, #2446, .T. ) ;
#21649=ORIENTED_EDGE ( 'NONE', *, *, #1006, .F. ) ;
#21651=CARTESIAN_POINT ( 'NONE',  ( 38.42058609394389634, 7.733997452150218166, 32.05199712042067262 ) ) ;
#21655=CARTESIAN_POINT ( 'NONE',  ( -23.72845085825479217, 12.99428747377815618, 47.94653096642124268 ) ) ;
#21665=DIRECTION ( 'NONE',  ( 0.000000000000000000, 0.000000000000000000, 1.000000000000000000 ) ) ;
#21671=ORIENTED_EDGE ( 'NONE', *, *, #7117, .F. ) ;
#21673=CARTESIAN_POINT ( 'NONE',  ( -32.02759086605583150, -18.14861398546997862, 34.50000000000000000 ) ) ;
#21681=ORIENTED_EDGE ( 'NONE', *, *, #22660, .F. ) ;
#21690=ORIENTED_EDGE ( 'NONE', *, *, #8427, .T. ) ;
#21703=CARTESIAN_POINT ( 'NONE',  ( 30.06732515731210142, 27.07630587620099050, 30.35442667510426062 ) ) ;
#21704=EDGE_CURVE ( 'NONE', #9483, #14021, #16634, .T. ) ;
#21707=AXIS2_PLACEMENT_3D ( 'NONE', #1412, #29798, #3126 ) ;
#21710=CARTESIAN_POINT ( 'NONE',  ( 32.28307784207223108, -8.475829241206289666, 37.38016955275583086 ) ) ;
#21712=ORIENTED_EDGE ( 'NONE', *, *, #12246, .F. ) ;
#21721=CARTESIAN_POINT ( 'NONE',  ( -17.79341399750137498, 34.33949722786772440, 34.50000000000000000 ) ) ;
#21727=CARTESIAN_POINT ( 'NONE',  ( -23.13391957319673864, -11.02874123662317984, 45.12930086386443662 ) ) ;
#21745=ORIENTED_EDGE ( 'NONE', *, *, #3267, .F. ) ;
#21765=CARTESIAN_POINT ( 'NONE',  ( -30.15176711667785980, -27.09037013813884798, 30.35400163365964943 ) ) ;
#21770=DIRECTION ( 'NONE',  ( 1.000000000000000000, 0.000000000000000000, -0.000000000000000000 ) ) ;
#21791=DIRECTION ( 'NONE',  ( -0.000000000000000000, -0.000000000000000000, 1.000000000000000000 ) ) ;
#21812=AXIS2_PLACEMENT_3D ( 'NONE', #2499, #28547, #19340 ) ;
#21816=CARTESIAN_POINT ( 'NONE',  ( 24.35970437652574816, -13.37404834226503958, -16.55003854064094426 ) ) ;
#21825=ORIENTED_EDGE ( 'NONE', *, *, #11116, .F. ) ;
#21835=ORIENTED_EDGE ( 'NONE', *, *, #1210, .F. ) ;
#21836=CARTESIAN_POINT ( 'NONE',  ( -4.375757216953428294E-15, -39.50000000000000000, 34.49999999999999289 ) ) ;
#21840=CYLINDRICAL_SURFACE ( 'NONE', #10473, 2.000000000000001776 ) ;
#21850=CARTESIAN_POINT ( 'NONE',  ( 23.62400240902268322, 9.724154461249522541, 49.47829057475696857 ) ) ;
#21852=CARTESIAN_POINT ( 'NONE',  ( 32.28307784207223108, 8.475829241206289666, 41.62281023987511475 ) ) ;
#21859=CARTESIAN_POINT ( 'NONE',  ( 24.44496207165490276, 7.595930209050162141, 49.40206402021032517 ) ) ;
#21870=DIRECTION ( 'NONE',  ( -0.000000000000000000, -0.000000000000000000, -1.000000000000000000 ) ) ;
#21871=CARTESIAN_POINT ( 'NONE',  ( 35.12146917884712138, 13.20565518866672505, 37.49999999998515676 ) ) ;
#21874=VECTOR ( 'NONE', #4349, 1000.000000000000000 ) ;
#21881=ORIENTED_EDGE ( 'NONE', *, *, #21704, .T. ) ;
#21887=CARTESIAN_POINT ( 'NONE',  ( -13.79366593457946344, 36.54982519354243209, 34.50000000000000000 ) ) ;
#21920=CARTESIAN_POINT ( 'NONE',  ( -30.34931995752844358, -22.03541669038290607, 37.50000000004472867 ) ) ;
#21922=CARTESIAN_POINT ( 'NONE',  ( -24.44496207165490276, 7.595930209050158588, 49.40206402021040333 ) ) ;
#21930=EDGE_CURVE ( 'NONE', #1203, #8258, #4362, .T. ) ;
#21946=ORIENTED_EDGE ( 'NONE', *, *, #22309, .F. ) ;
#21956=EDGE_CURVE ( 'NONE', #26848, #19902, #2884, .T. ) ;
#21963=CARTESIAN_POINT ( 'NONE',  ( 27.29267191310605156, 30.38807181596501650, 30.00869227221143731 ) ) ;
#21968=CARTESIAN_POINT ( 'NONE',  ( -31.29189664795533332, -25.39986983782039687, 30.52943660264045178 ) ) ;
#22004=CARTESIAN_POINT ( 'NONE',  ( 1.015311529865299489, 39.50000000000000000, 34.49999999999999289 ) ) ;
#22005=CARTESIAN_POINT ( 'NONE',  ( -35.13669516613692423, -8.778141986582063794, 34.58384122122906490 ) ) ;
#22006=CARTESIAN_POINT ( 'NONE',  ( 31.57476163834523675, 15.10795358447670189, 39.99718304312875716 ) ) ;
#22021=CARTESIAN_POINT ( 'NONE',  ( -25.07950435457407323, -11.50806656539752737, -16.55003854064094426 ) ) ;
#22041=DIRECTION ( 'NONE',  ( -0.9329908884337543284, -0.3598999890241648125, 0.000000000000000000 ) ) ;
#22068=CARTESIAN_POINT ( 'NONE',  ( -29.59797164802278857, -23.03477555636723650, 37.49999999995527133 ) ) ;
#22080=DIRECTION ( 'NONE',  ( -0.000000000000000000, -0.000000000000000000, 1.000000000000000000 ) ) ;
#22084=ORIENTED_EDGE ( 'NONE', *, *, #7279, .T. ) ;
#22090=EDGE_CURVE ( 'NONE', #10953, #20218, #24849, .T. ) ;
#22093=DIRECTION ( 'NONE',  ( -0.000000000000000000, -0.000000000000000000, -1.000000000000000000 ) ) ;
#22095=ORIENTED_EDGE ( 'NONE', *, *, #5362, .F. ) ;
#22096=CARTESIAN_POINT ( 'NONE',  ( -6.191185452821632573, -38.91708858248148317, 27.50000000000000000 ) ) ;
#22109=CARTESIAN_POINT ( 'NONE',  ( 6.176953700987930951, 38.93706494759733516, 27.50000000000000355 ) ) ;
#22113=CARTESIAN_POINT ( 'NONE',  ( 28.56150147175966936, 28.94728505588477674, 30.15884368954713679 ) ) ;
#22117=CARTESIAN_POINT ( 'NONE',  ( -31.36844279130544777, 25.28729038194961731, 30.54136519211768430 ) ) ;
#22118=CARTESIAN_POINT ( 'NONE',  ( 77.99999999999998579, 42.50000000000000711, 32.26246401786215756 ) ) ;
#22122=CARTESIAN_POINT ( 'NONE',  ( 33.53502205450880069, -14.39784139885291836, 34.49999999999999289 ) ) ;
#22130=EDGE_CURVE ( 'NONE', #30416, #11554, #22979, .T. ) ;
#22151=CARTESIAN_POINT ( 'NONE',  ( -32.60829997825918980, 13.18983524832148291, 39.84356070656662041 ) ) ;
#22153=CARTESIAN_POINT ( 'NONE',  ( -25.18466322232233523, 6.657711795334218863, 44.70772167919928108 ) ) ;
#22159=AXIS2_PLACEMENT_3D ( 'NONE', #4425, #16431, #13940 ) ;
#22160=CARTESIAN_POINT ( 'NONE',  ( -27.03943647958860552, 26.20092231554396633, 34.80090346875805096 ) ) ;
#22164=CARTESIAN_POINT ( 'NONE',  ( -25.18096005886327760, -6.640581704039637323, 48.95928115109028766 ) ) ;
#22166=DIRECTION ( 'NONE',  ( 0.000000000000000000, 0.000000000000000000, 1.000000000000000000 ) ) ;
#22186=ADVANCED_FACE ( 'NONE', ( #627 ), #28878, .F. ) ;
#22190=CARTESIAN_POINT ( 'NONE',  ( -8.523310919002204500, 38.38027722185356083, 34.49999999999998579 ) ) ;
#22193=CARTESIAN_POINT ( 'NONE',  ( -30.53339558441486190, 7.800891647352838909, 39.24389099736758624 ) ) ;
#22198=( NAMED_UNIT ( * ) SI_UNIT ( $, .STERADIAN. ) SOLID_ANGLE_UNIT ( ) );
#22204=DIRECTION ( 'NONE',  ( 0.9898434871385290990, -0.1411469255096601816, 0.01695335921306606250 ) ) ;
#22209=AXIS2_PLACEMENT_3D ( 'NONE', #12009, #4363, #11694 ) ;
#22225=CARTESIAN_POINT ( 'NONE',  ( -33.31528697581643428, -22.10504849272555106, 30.86792493716536612 ) ) ;
#22232=FACE_OUTER_BOUND ( 'NONE', #4593, .T. ) ;
#22238=VECTOR ( 'NONE', #28617, 1000.000000000000000 ) ;
#22256=CARTESIAN_POINT ( 'NONE',  ( -6.804986885018592169, -38.79337642873097991, 27.50000000000000355 ) ) ;
#22268=CARTESIAN_POINT ( 'NONE',  ( 14.89790177301713392, 39.30146707257869565, 29.12506352215398664 ) ) ;
#22273=CARTESIAN_POINT ( 'NONE',  ( -29.04471618533923305, -28.48400268535028346, 30.20750335454674129 ) ) ;
#22275=EDGE_CURVE ( 'NONE', #7455, #18044, #29290, .T. ) ;
#22276=CARTESIAN_POINT ( 'NONE',  ( -29.61203839202723032, -15.40012917324033381, 37.38016955275590192 ) ) ;
#22277=ORIENTED_EDGE ( 'NONE', *, *, #2103, .F. ) ;
#22300=EDGE_LOOP ( 'NONE', ( #26284, #19275, #21881, #10595 ) ) ;
#22305=CARTESIAN_POINT ( 'NONE',  ( 32.14097302481091134, -14.40131566728160273, 35.53783135158875695 ) ) ;
#22309=EDGE_CURVE ( 'NONE', #22753, #6144, #9230, .T. ) ;
#22312=CARTESIAN_POINT ( 'NONE',  ( 15.63826127963997870, 35.59355150539998647, 34.50000000000000000 ) ) ;
#22316=CARTESIAN_POINT ( 'NONE',  ( -2.338573377552018773, 39.50000000000000711, 27.50000000000000355 ) ) ;
#22325=CARTESIAN_POINT ( 'NONE',  ( 33.47438960496221227, 10.94461781313380477, 35.53941315612136975 ) ) ;
#22336=CARTESIAN_POINT ( 'NONE',  ( 77.99999999999998579, 42.50000000000000000, 27.50000000000000711 ) ) ;
#22338=CARTESIAN_POINT ( 'NONE',  ( 15.37842778815315725, 39.08494192275733781, 34.54087420883106319 ) ) ;
#22346=ADVANCED_FACE ( 'NONE', ( #5264, #10092, #10242 ), #29339, .F. ) ;
#22351=CARTESIAN_POINT ( 'NONE',  ( -19.07766892062203468, 33.49890683909209343, 34.49999999999998579 ) ) ;
#22376=CARTESIAN_POINT ( 'NONE',  ( -31.89304216768361400, 14.79375299452194703, 35.60059606544055555 ) ) ;
#22378=CARTESIAN_POINT ( 'NONE',  ( 5.965445004520304018, -42.10621517464141306, 34.60264052001484458 ) ) ;
#22390=CARTESIAN_POINT ( 'NONE',  ( -37.12542188692624734, 5.327348916628460884, 37.50000000001456613 ) ) ;
#22404=CARTESIAN_POINT ( 'NONE',  ( 36.00000000000000000, -1.546978760965586295E-11, 34.75735931288068059 ) ) ;
#22413=CARTESIAN_POINT ( 'NONE',  ( -4.375757216953428294E-15, -39.50000000000000000, 27.50000000000000355 ) ) ;
#22427=CARTESIAN_POINT ( 'NONE',  ( 34.59464071930022300, -19.79227917861567221, 31.10398916234817079 ) ) ;
#22431=CARTESIAN_POINT ( 'NONE',  ( -38.39051948279409743, 7.594952977269135097, 32.04396099389172292 ) ) ;
#22451=ORIENTED_EDGE ( 'NONE', *, *, #26013, .F. ) ;
#22455=CARTESIAN_POINT ( 'NONE',  ( 29.61203839202725518, -15.40012917324033381, 37.38016955275580244 ) ) ;
#22459=CARTESIAN_POINT ( 'NONE',  ( 33.55239377822428537, 10.10392708029668185, 39.95942412019666534 ) ) ;
#22462=CARTESIAN_POINT ( 'NONE',  ( -28.55068628633582861, 24.19494186940698199, 34.80090346875805096 ) ) ;
#22473=B_SPLINE_CURVE_WITH_KNOTS ( 'NONE', 3,
 ( #11219, #21021, #18093, #18553, #3748, #6394, #13267, #1414, #20431, #25423, #8588, #4049, #8891, #18415 ),
 .UNSPECIFIED., .F., .F.,
 ( 4, 2, 2, 2, 2, 2, 4 ),
 ( 2.111164903073641426E-07, 0.0004668847526555942461, 0.0009335583888208811134, 0.001400232024986168035, 0.001866905661151454848, 0.002800252933482020451, 0.003733600205812585837 ),
 .UNSPECIFIED. ) ;
#22481=CARTESIAN_POINT ( 'NONE',  ( 25.41654339919795902, 6.509636863629522097, 44.52079389600188364 ) ) ;
#22503=ORIENTED_EDGE ( 'NONE', *, *, #5526, .T. ) ;
#22511=ORIENTED_EDGE ( 'NONE', *, *, #24384, .F. ) ;
#22512=CARTESIAN_POINT ( 'NONE',  ( -30.03865005752670214, 15.52610542268208604, 36.94359686637174178 ) ) ;
#22528=CARTESIAN_POINT ( 'NONE',  ( -4.272706734768129344, -37.25579118954082247, 37.50000000000000000 ) ) ;
#22549=CARTESIAN_POINT ( 'NONE',  ( 32.89824568090541845, -8.841523719485385513, 40.93443584516763423 ) ) ;
#22575=CARTESIAN_POINT ( 'NONE',  ( -26.11179934312166395, 14.04991663536888780, 41.10667063058299675 ) ) ;
#22591=ORIENTED_EDGE ( 'NONE', *, *, #26550, .F. ) ;
#22592=ORIENTED_EDGE ( 'NONE', *, *, #10939, .T. ) ;
#22593=DIRECTION ( 'NONE',  ( 0.9329908884337537733, -0.3598999890241659783, 0.000000000000000000 ) ) ;
#22602=CARTESIAN_POINT ( 'NONE',  ( 22.49999999999992184, 1.663324310589599759E-14, 62.49999999999999289 ) ) ;
#22622=LINE ( 'NONE', #15930, #11747 ) ;
#22637=CARTESIAN_POINT ( 'NONE',  ( -32.49060333908415288, 8.555881924488323520, 41.40175883617482100 ) ) ;
#22654=ORIENTED_EDGE ( 'NONE', *, *, #8631, .F. ) ;
#22660=EDGE_CURVE ( 'NONE', #12760, #30101, #27711, .T. ) ;
#22662=CARTESIAN_POINT ( 'NONE',  ( 24.44496207165490631, -7.595930209050163029, -16.55003854064094426 ) ) ;
#22665=CARTESIAN_POINT ( 'NONE',  ( -30.50257113119998209, 15.54031451041691270, 36.52435908487349536 ) ) ;
#22667=CARTESIAN_POINT ( 'NONE',  ( -3.741133385587110283, -42.33143344558632748, 28.85421604109468063 ) ) ;
#22675=CARTESIAN_POINT ( 'NONE',  ( -5.433041902549405222, -37.12271733102753046, 37.49999999999359801 ) ) ;
#22679=CARTESIAN_POINT ( 'NONE',  ( 32.06827542805550735, -14.53851282002520406, 39.79035104390192146 ) ) ;
#22680=CARTESIAN_POINT ( 'NONE',  ( -24.03448224033878944, 8.660042335149837456, 45.23564988763775574 ) ) ;
#22682=CARTESIAN_POINT ( 'NONE',  ( 6.601643239663004076E-16, 42.50000000000000000, 28.83974596215562514 ) ) ;
#22724=EDGE_CURVE ( 'NONE', #3185, #26303, #30806, .T. ) ;
#22736=VERTEX_POINT ( 'NONE', #9603 ) ;
#22740=CARTESIAN_POINT ( 'NONE',  ( 35.76481447503398670, -5.202797454133663457, 34.80090346875810070 ) ) ;
#22752=CARTESIAN_POINT ( 'NONE',  ( 23.21352257770656990, 10.78826658734920230, 49.40206402021032517 ) ) ;
#22753=VERTEX_POINT ( 'NONE', #14258 ) ;
#22769=B_SPLINE_CURVE_WITH_KNOTS ( 'NONE', 3,
 ( #27899, #23495, #28502, #25548, #13553, #11515, #26008, #28184, #8867, #21145, #23032, #28357, #16491, #4636 ),
 .UNSPECIFIED., .F., .F.,
 ( 4, 2, 2, 2, 2, 2, 4 ),
 ( 2.108610145937280049E-07, 0.0004867403503157841311, 0.0009732698396169746011, 0.001459799328918164746, 0.001946328818219355324, 0.002919387796821722603, 0.003892446775424090316 ),
 .UNSPECIFIED. ) ;
#22774=CARTESIAN_POINT ( 'NONE',  ( -17.94248964168179938, -34.33858135081683827, 27.50000000000001066 ) ) ;
#22784=ORIENTED_EDGE ( 'NONE', *, *, #9963, .F. ) ;
#22788=DIRECTION ( 'NONE',  ( 1.000000000000000000, 0.000000000000000000, 0.000000000000000000 ) ) ;
#22800=AXIS2_PLACEMENT_3D ( 'NONE', #10862, #8533, #6178 ) ;
#22803=ORIENTED_EDGE ( 'NONE', *, *, #9033, .F. ) ;
#22827=LINE ( 'NONE', #22662, #5637 ) ;
#22832=CARTESIAN_POINT ( 'NONE',  ( 0.4781620243103129053, -42.50348742054170970, 34.61334324197476775 ) ) ;
#22847=CARTESIAN_POINT ( 'NONE',  ( -29.61203839202723032, -15.40012917324033381, 41.62281023987518580 ) ) ;
#22859=CARTESIAN_POINT ( 'NONE',  ( -37.50000000000005684, 9.285362311011880811E-15, 37.50000000000000000 ) ) ;
#22860=CARTESIAN_POINT ( 'NONE',  ( 32.28307784207223108, -8.475829241206289666, 41.62281023987511475 ) ) ;
#22862=CIRCLE ( 'NONE', #9426, 37.50000000000001421 ) ;
#22868=ORIENTED_EDGE ( 'NONE', *, *, #22724, .F. ) ;
#22873=VERTEX_POINT ( 'NONE', #14890 ) ;
#22891=ADVANCED_FACE ( 'NONE', ( #7885 ), #7309, .T. ) ;
#22895=ORIENTED_EDGE ( 'NONE', *, *, #11639, .T. ) ;
#22898=CARTESIAN_POINT ( 'NONE',  ( 35.99999999999999289, -2.601438916704202242, 27.50000000000001066 ) ) ;
#22907=EDGE_CURVE ( 'NONE', #14013, #29295, #20309, .T. ) ;
#22908=DIRECTION ( 'NONE',  ( -0.000000000000000000, -0.000000000000000000, 1.000000000000000000 ) ) ;
#22938=LINE ( 'NONE', #20901, #10639 ) ;
#22946=DIRECTION ( 'NONE',  ( -0.000000000000000000, -0.000000000000000000, 1.000000000000000000 ) ) ;
#22947=VERTEX_POINT ( 'NONE', #6718 ) ;
#22963=CARTESIAN_POINT ( 'NONE',  ( 32.19782014694308003, -14.25394737442115201, 39.78814634291934738 ) ) ;
#22971=EDGE_CURVE ( 'NONE', #4164, #14021, #7692, .T. ) ;
#22973=ADVANCED_FACE ( 'NONE', ( #4082 ), #1448, .F. ) ;
#22978=CARTESIAN_POINT ( 'NONE',  ( 29.48815749055103552, -23.29943950550710952, 37.50000000016476775 ) ) ;
#22979=B_SPLINE_CURVE_WITH_KNOTS ( 'NONE', 3,
 ( #17201, #26724, #24378, #12541 ),
 .UNSPECIFIED., .F., .F.,
 ( 4, 4 ),
 ( 3.022186913405034649E-07, 0.007932103869840197510 ),
 .UNSPECIFIED. ) ;
#22988=CARTESIAN_POINT ( 'NONE',  ( -10.03589362353479686, -36.13692893856508448, 37.49999999997990585 ) ) ;
#22993=CARTESIAN_POINT ( 'NONE',  ( 31.57687401261851434, -15.10620312102103213, 39.99603010801624237 ) ) ;
#22995=ORIENTED_EDGE ( 'NONE', *, *, #4253, .F. ) ;
#22999=CARTESIAN_POINT ( 'NONE',  ( 32.19782014694307293, 14.25394737442116444, 35.54550565580007770 ) ) ;
#23007=ORIENTED_EDGE ( 'NONE', *, *, #21603, .T. ) ;
#23011=DIRECTION ( 'NONE',  ( -0.000000000000000000, -0.000000000000000000, 1.000000000000000000 ) ) ;
#23012=ORIENTED_EDGE ( 'NONE', *, *, #22275, .F. ) ;
#23021=CARTESIAN_POINT ( 'NONE',  ( -0.5205051961121548443, 42.60095040672530331, 34.61591466868899403 ) ) ;
#23031=CARTESIAN_POINT ( 'NONE',  ( 33.42393154775842135, -22.05663106644447424, 30.87484722992571307 ) ) ;
#23032=CARTESIAN_POINT ( 'NONE',  ( 26.12047388987419794, -6.311255530320351248, 48.12792051007059513 ) ) ;
#23039=CARTESIAN_POINT ( 'NONE',  ( 23.69412710310940540, -29.84645176427128987, 34.80090346875809360 ) ) ;
#23055=ORIENTED_EDGE ( 'NONE', *, *, #13004, .F. ) ;
#23059=ORIENTED_EDGE ( 'NONE', *, *, #29111, .T. ) ;
#23060=VERTEX_POINT ( 'NONE', #30277 ) ;
#23067=CARTESIAN_POINT ( 'NONE',  ( -28.55068628633583216, -24.19494186940697134, 27.50000000000000355 ) ) ;
#23068=CYLINDRICAL_SURFACE ( 'NONE', #10332, 1.999999999999998224 ) ;
#23072=EDGE_CURVE ( 'NONE', #19902, #18416, #8616, .T. ) ;
#23084=CARTESIAN_POINT ( 'NONE',  ( 32.19782014694307293, 14.25394737442116444, 39.78814634291936159 ) ) ;
#23096=CARTESIAN_POINT ( 'NONE',  ( -34.70577939416727276, 10.49309206033987785, 34.49999999999999289 ) ) ;
#23121=LINE ( 'NONE', #11282, #7076 ) ;
#23130=CARTESIAN_POINT ( 'NONE',  ( 38.48713303109791894, -7.360220187875558651, 35.02549194227622564 ) ) ;
#23139=CARTESIAN_POINT ( 'NONE',  ( -10.59559327413201046, -40.90840839550211427, 28.97918858187435021 ) ) ;
#23141=CARTESIAN_POINT ( 'NONE',  ( -32.14095006730909176, -14.40137518142634576, 39.78046893946850560 ) ) ;
#23171=FACE_OUTER_BOUND ( 'NONE', #30819, .T. ) ;
#23194=B_SPLINE_CURVE_WITH_KNOTS ( 'NONE', 3,
 ( #1526, #14405, #4012, #2398, #18208, #15701, #15866, #29915, #28451, #27722, #21095, #9262, #10882, #14082, #23590, #11035 ),
 .UNSPECIFIED., .F., .F.,
 ( 4, 2, 2, 2, 2, 2, 2, 4 ),
 ( 2.980374332640320740E-07, 0.0009280375596593466898, 0.001391907320772395144, 0.001855777081885443599, 0.002319646842998492053, 0.002783516604111547880, 0.003247386365224604141, 0.003711256126337660836 ),
 .UNSPECIFIED. ) ;
#23219=CARTESIAN_POINT ( 'NONE',  ( -27.03943647958861263, -26.20092231554396278, 27.50000000000000355 ) ) ;
#23236=CARTESIAN_POINT ( 'NONE',  ( -16.53781638505575557, 35.10828276421680272, 27.49999999999999645 ) ) ;
#23248=ORIENTED_EDGE ( 'NONE', *, *, #587, .F. ) ;
#23278=ADVANCED_BREP_SHAPE_REPRESENTATION ( '', ( #3432, #7396 ), #15375 ) ;
#23284=CARTESIAN_POINT ( 'NONE',  ( 17.34672660037420044, -33.26777931996199555, 37.50000000003682032 ) ) ;
#23294=ADVANCED_FACE ( 'NONE', ( #15736 ), #8726, .F. ) ;
#23296=ADVANCED_FACE ( 'NONE', ( #6681 ), #16196, .T. ) ;
#23299=CARTESIAN_POINT ( 'NONE',  ( -24.58208797071834439, -7.298293523701636865, 45.11515778355300199 ) ) ;
#23304=CARTESIAN_POINT ( 'NONE',  ( 31.10500197267672462, -15.38309308716404722, 40.29910134388152443 ) ) ;
#23307=EDGE_CURVE ( 'NONE', #17402, #1784, #10216, .T. ) ;
#23308=CARTESIAN_POINT ( 'NONE',  ( 23.21076833940160000, 12.23288291591659771, 44.52046879181326489 ) ) ;
#23323=VERTEX_POINT ( 'NONE', #10923 ) ;
#23326=EDGE_CURVE ( 'NONE', #2857, #10874, #13611, .T. ) ;
#23360=CARTESIAN_POINT ( 'NONE',  ( 32.31576317091162309, 17.59561277345964214, 27.49999999999999645 ) ) ;
#23369=CARTESIAN_POINT ( 'NONE',  ( 23.26155266345718431, 12.35118985415806847, 48.66282223823449726 ) ) ;
#23389=CARTESIAN_POINT ( 'NONE',  ( 24.03448224033878944, -8.660042335149841009, 45.23564988763768469 ) ) ;
#23400=CARTESIAN_POINT ( 'NONE',  ( -2.468401054669552952, 39.50000000000001421, 27.50000000000001421 ) ) ;
#23401=CARTESIAN_POINT ( 'NONE',  ( 23.20389136007291953, -12.24563090271730736, 48.76343458319715296 ) ) ;
#23432=CARTESIAN_POINT ( 'NONE',  ( 31.98172739339260673, -24.47984296869126908, 34.62180873253410596 ) ) ;
#23447=CARTESIAN_POINT ( 'NONE',  ( 29.61203839202725518, -15.40012917324033381, 41.62281023987508632 ) ) ;
#23452=CARTESIAN_POINT ( 'NONE',  ( 0.000000000000000000, 39.50000000000000000, 34.49999999999999289 ) ) ;
#23480=CARTESIAN_POINT ( 'NONE',  ( 33.42925964089141644, -11.06161099612213228, -16.55003854064094426 ) ) ;
#23483=CARTESIAN_POINT ( 'NONE',  ( -15.76609453206417832, 34.02993354821598615, 37.50000000001164580 ) ) ;
#23488=CARTESIAN_POINT ( 'NONE',  ( 33.42925964089140933, 11.06161099612213405, 35.54550565580007060 ) ) ;
#23495=CARTESIAN_POINT ( 'NONE',  ( 24.50429677314015819, -7.442113211156453190, 49.39104550111578362 ) ) ;
#23504=CARTESIAN_POINT ( 'NONE',  ( 0.000000000000000000, 39.50000000000000000, 27.50000000000000355 ) ) ;
#23511=DIRECTION ( 'NONE',  ( -0.000000000000000000, -0.000000000000000000, 1.000000000000000000 ) ) ;
#23517=ORIENTED_EDGE ( 'NONE', *, *, #25695, .T. ) ;
#23529=CARTESIAN_POINT ( 'NONE',  ( -23.15749938697695143, 12.07134380388759709, 48.88521798569314569 ) ) ;
#23543=CARTESIAN_POINT ( 'NONE',  ( -18.12723876908564691, 34.13071258496300686, 27.50000000000000711 ) ) ;
#23545=ORIENTED_EDGE ( 'NONE', *, *, #8977, .T. ) ;
#23557=CARTESIAN_POINT ( 'NONE',  ( 34.90527075214175312, -9.744570251167933961, 27.50000000000000711 ) ) ;
#23575=FACE_OUTER_BOUND ( 'NONE', #13789, .T. ) ;
#23582=CARTESIAN_POINT ( 'NONE',  ( 28.09938986509257930, 29.50836898064226688, 34.53879572982188506 ) ) ;
#23588=ORIENTED_EDGE ( 'NONE', *, *, #19268, .F. ) ;
#23590=CARTESIAN_POINT ( 'NONE',  ( -32.14095006730909176, -14.40137518142634576, 35.53782825234922171 ) ) ;
#23594=AXIS2_PLACEMENT_3D ( 'NONE', #14929, #21791, #7761 ) ;
#23611=CARTESIAN_POINT ( 'NONE',  ( 32.89824568090541845, -8.841523719485381960, 36.69179515804835034 ) ) ;
#23627=CARTESIAN_POINT ( 'NONE',  ( -37.01201912122522231, 13.45809432592687038, 31.66270403581487258 ) ) ;
#23648=CARTESIAN_POINT ( 'NONE',  ( 11.52197458429827037, 37.50933785548059518, 27.50000000000000355 ) ) ;
#23675=CARTESIAN_POINT ( 'NONE',  ( -7.658030750032036593, -41.69611546128646751, 28.90941362898500699 ) ) ;
#23681=CARTESIAN_POINT ( 'NONE',  ( 10.94975753521667095, -37.63148039617637153, 34.49999999999998579 ) ) ;
#23697=CARTESIAN_POINT ( 'NONE',  ( -15.65263381497855200, -35.63608703567959424, 34.50000000000000000 ) ) ;
#23709=CARTESIAN_POINT ( 'NONE',  ( 24.34596477403963277, 29.10061797482480017, 27.50000000000001066 ) ) ;
#23718=LINE ( 'NONE', #4401, #18797 ) ;
#23724=CARTESIAN_POINT ( 'NONE',  ( -33.42925964089141644, 11.06161099612212695, -16.55003854064094426 ) ) ;
#23735=CARTESIAN_POINT ( 'NONE',  ( 37.46474186269768580, -2.090463118055147618, 37.49999999995337419 ) ) ;
#23739=ORIENTED_EDGE ( 'NONE', *, *, #14349, .T. ) ;
#23792=CARTESIAN_POINT ( 'NONE',  ( -29.09978263823398237, 28.32965845976518082, 30.22324450238831872 ) ) ;
#23794=CARTESIAN_POINT ( 'NONE',  ( -27.86235613436986114, -14.72519157938688750, 43.48653168448685591 ) ) ;
#23831=PRODUCT_DEFINITION_FORMATION_WITH_SPECIFIED_SOURCE ( 'ANY', '', #26888, .NOT_KNOWN. ) ;
#23834=VECTOR ( 'NONE', #16494, 1000.000000000000000 ) ;
#23861=CARTESIAN_POINT ( 'NONE',  ( -35.78592255317990123, -4.958958154555994646, 27.50000000000000355 ) ) ;
#23865=CARTESIAN_POINT ( 'NONE',  ( -1.025177369996997268, -39.49999999999999289, 34.49999999999998579 ) ) ;
#23870=ORIENTED_EDGE ( 'NONE', *, *, #28636, .T. ) ;
#23878=CARTESIAN_POINT ( 'NONE',  ( 27.62938074698936219, -25.35013884327572242, 27.49999999999999645 ) ) ;
#23883=CARTESIAN_POINT ( 'NONE',  ( -31.10500197267670330, 15.38309308716404900, 40.29910134388162390 ) ) ;
#23885=ADVANCED_FACE ( 'NONE', ( #3479 ), #24987, .F. ) ;
#23889=PLANE ( 'NONE',  #30739 ) ;
#23899=VERTEX_POINT ( 'NONE', #6582 ) ;
#23901=CARTESIAN_POINT ( 'NONE',  ( 37.45995770769625466, 1.852643206688098232, 37.49999999997684341 ) ) ;
#23903=ORIENTED_EDGE ( 'NONE', *, *, #28194, .F. ) ;
#23926=EDGE_CURVE ( 'NONE', #20218, #20928, #1309, .T. ) ;
#23948=CARTESIAN_POINT ( 'NONE',  ( -18.10334121439571931, 37.65254011239409948, 34.52361733454125670 ) ) ;
#23950=CARTESIAN_POINT ( 'NONE',  ( -26.11179934312166040, -14.04991663536888780, 45.34931131770226642 ) ) ;
#23952=CARTESIAN_POINT ( 'NONE',  ( 32.90011853910910844, 8.843064278303863546, 36.68958760228017013 ) ) ;
#23964=CYLINDRICAL_SURFACE ( 'NONE', #14764, 1.999999999999998224 ) ;
#23977=CARTESIAN_POINT ( 'NONE',  ( -4.163336342344337027E-14, 1.387778780781445676E-14, 51.25735931288069480 ) ) ;
#23983=CARTESIAN_POINT ( 'NONE',  ( 21.62412008219442683, 35.47471372268120859, 29.49052918880962437 ) ) ;
#23996=ORIENTED_EDGE ( 'NONE', *, *, #1006, .T. ) ;
#24017=AXIS2_PLACEMENT_3D ( 'NONE', #11843, #13725, #18867 ) ;
#24028=CARTESIAN_POINT ( 'NONE',  ( -31.22647667302024388, 15.32805873036034505, 40.21452297286847966 ) ) ;
#24046=CARTESIAN_POINT ( 'NONE',  ( 22.33591402143825277, 34.95758375282650832, 34.50523401540510804 ) ) ;
#24050=CARTESIAN_POINT ( 'NONE',  ( -23.21352257770656990, -10.78826658734919519, -16.55003854064094426 ) ) ;
#24083=B_SPLINE_CURVE_WITH_KNOTS ( 'NONE', 3,
 ( #28775, #2733, #8035, #17538 ),
 .UNSPECIFIED., .F., .F.,
 ( 4, 4 ),
 ( 2.143643656964903906E-07, 0.003421830178490235450 ),
 .UNSPECIFIED. ) ;
#24093=FACE_OUTER_BOUND ( 'NONE', #26850, .T. ) ;
#24103=CARTESIAN_POINT ( 'NONE',  ( -25.60051251894998003, 32.07260926886260677, 34.51546816935509554 ) ) ;
#24128=EDGE_LOOP ( 'NONE', ( #15432, #5237, #13093, #10745 ) ) ;
#24132=CARTESIAN_POINT ( 'NONE',  ( -25.88604317058895532, 6.345278376181626712, 48.34797144667707869 ) ) ;
#24134=ADVANCED_FACE ( 'NONE', ( #14513 ), #21840, .F. ) ;
#24135=CARTESIAN_POINT ( 'NONE',  ( 23.15419545472248686, -10.94206393902796925, 45.14840622133245063 ) ) ;
#24144=CARTESIAN_POINT ( 'NONE',  ( -27.37266257347463494, -30.39118854371129075, 30.00740378720065493 ) ) ;
#24149=CARTESIAN_POINT ( 'NONE',  ( 31.11989886121315863, -19.96255629701192902, 34.50000000000000000 ) ) ;
#24151=CYLINDRICAL_SURFACE ( 'NONE', #8823, 2.000000000000001776 ) ;
#24161=CARTESIAN_POINT ( 'NONE',  ( -27.81955209195762180, -25.07120904824700958, 34.50000000000000711 ) ) ;
#24169=DIRECTION ( 'NONE',  ( -0.000000000000000000, -0.000000000000000000, 1.000000000000000000 ) ) ;
#24174=CARTESIAN_POINT ( 'NONE',  ( -23.21352257770656990, 10.78826658734919519, -16.55003854064094426 ) ) ;
#24180=CARTESIAN_POINT ( 'NONE',  ( 33.56327786402390245, 10.46063060613185414, 39.84455206157484497 ) ) ;
#24184=AXIS2_PLACEMENT_3D ( 'NONE', #11318, #4280, #18494 ) ;
#24185=FACE_OUTER_BOUND ( 'NONE', #30609, .T. ) ;
#24194=CARTESIAN_POINT ( 'NONE',  ( 38.72184494665977184, 5.684323948905047885, 32.14431142672166430 ) ) ;
#24214=FACE_OUTER_BOUND ( 'NONE', #772, .T. ) ;
#24232=CARTESIAN_POINT ( 'NONE',  ( -23.15749938697695143, 12.07134380388760242, 44.64257729857385470 ) ) ;
#24245=SHAPE_DEFINITION_REPRESENTATION ( #28600, #19685 ) ;
#24246=EDGE_CURVE ( 'NONE', #19828, #17963, #1702, .T. ) ;
#24253=CARTESIAN_POINT ( 'NONE',  ( -24.44496207165490276, -7.595930209050158588, 45.15942333309111234 ) ) ;
#24256=CARTESIAN_POINT ( 'NONE',  ( -23.07950435457351190, 11.50806656539842798, 44.96784366550151191 ) ) ;
#24259=CARTESIAN_POINT ( 'NONE',  ( -31.76737364660611718, -19.96634320003312268, 37.49999999999806022 ) ) ;
#24262=CARTESIAN_POINT ( 'NONE',  ( -23.62400240902268322, 9.724154461249517212, 49.47829057475703962 ) ) ;
#24264=CARTESIAN_POINT ( 'NONE',  ( 32.60641126234700238, 8.625635766581060793, 37.02940160128806468 ) ) ;
#24277=CARTESIAN_POINT ( 'NONE',  ( -4.776122516674677878E-15, -42.50000000000000000, 27.50000000000000355 ) ) ;
#24310=CARTESIAN_POINT ( 'NONE',  ( -25.60834283456843963, 32.16668900101505812, 29.82420505145413969 ) ) ;
#24344=CARTESIAN_POINT ( 'NONE',  ( 32.01792732732114644, 18.17191813560462066, 34.49999999999999289 ) ) ;
#24348=CARTESIAN_POINT ( 'NONE',  ( 24.86084284002701850, 6.930828199065646622, 49.19141369485814863 ) ) ;
#24351=EDGE_CURVE ( 'NONE', #29295, #30416, #22473, .T. ) ;
#24369=CARTESIAN_POINT ( 'NONE',  ( -23.07950435457407679, -11.50806656539752737, 44.96784366550136980 ) ) ;
#24376=ORIENTED_EDGE ( 'NONE', *, *, #4412, .F. ) ;
#24378=CARTESIAN_POINT ( 'NONE',  ( -28.78283879316666471, -7.125616703334840984, 45.34931131770227353 ) ) ;
#24379=CARTESIAN_POINT ( 'NONE',  ( -7.031646814991431071, 38.74271536321815290, 34.49999999999999289 ) ) ;
#24382=CARTESIAN_POINT ( 'NONE',  ( -28.78283879316666471, 7.125616703334840984, 41.10667063058299675 ) ) ;
#24384=EDGE_CURVE ( 'NONE', #17083, #6797, #1039, .T. ) ;
#24402=ORIENTED_EDGE ( 'NONE', *, *, #10521, .F. ) ;
#24407=EDGE_CURVE ( 'NONE', #22736, #2857, #1280, .T. ) ;
#24412=CARTESIAN_POINT ( 'NONE',  ( -31.71888454229558363, -24.74171469661772704, 34.61963941082733243 ) ) ;
#24419=LINE ( 'NONE', #9623, #3389 ) ;
#24425=CARTESIAN_POINT ( 'NONE',  ( -26.31094384852241319, -8.315730187098489878, -16.55003854064094426 ) ) ;
#24442=CARTESIAN_POINT ( 'NONE',  ( -12.15241004504941991, -37.27483646721038468, 27.50000000000000000 ) ) ;
#24452=CARTESIAN_POINT ( 'NONE',  ( 23.07500649350761179, -11.56036165373734725, 44.94877300775547013 ) ) ;
#24454=CARTESIAN_POINT ( 'NONE',  ( 35.79322151885497760, -4.895449333909911438, 27.50000000000000711 ) ) ;
#24458=CARTESIAN_POINT ( 'NONE',  ( 39.00445379423575787, 0.06697950101438043813, 32.23359341845904424 ) ) ;
#24463=CARTESIAN_POINT ( 'NONE',  ( -32.98872764523831336, -22.67896170318111970, 30.80968328952752699 ) ) ;
#24465=CARTESIAN_POINT ( 'NONE',  ( -27.86235613436986114, -14.72519157938688750, 39.24389099736757203 ) ) ;
#24468=CARTESIAN_POINT ( 'NONE',  ( 29.81396013349119301, -22.14051264938663266, 34.49999999999999289 ) ) ;
#24491=AXIS2_PLACEMENT_3D ( 'NONE', #6513, #4165, #18525 ) ;
#24492=CARTESIAN_POINT ( 'NONE',  ( -24.75800239156184546, 7.045788922043114688, 45.01673140503407211 ) ) ;
#24497=CARTESIAN_POINT ( 'NONE',  ( 2.034297646570668583, 39.45293230050472033, 34.50000000000000000 ) ) ;
#24498=CARTESIAN_POINT ( 'NONE',  ( -17.94248964168179938, 34.33858135081683827, 34.80090346875804386 ) ) ;
#24502=CARTESIAN_POINT ( 'NONE',  ( -26.81368379037235172, -6.366017791192966513, 47.44099319977362939 ) ) ;
#24510=AXIS2_PLACEMENT_3D ( 'NONE', #6316, #15986, #3681 ) ;
#24529=CARTESIAN_POINT ( 'NONE',  ( -6.533353553387044599, 38.84762322035204818, 34.49999999999999289 ) ) ;
#24550=CARTESIAN_POINT ( 'NONE',  ( 2.548218919432729823, -42.41581599557042637, 34.61094837024117510 ) ) ;
#24562=CARTESIAN_POINT ( 'NONE',  ( -36.11265399167034218, -10.12638981614433931, 37.50000000003317524 ) ) ;
#24572=CARTESIAN_POINT ( 'NONE',  ( 31.10273980501928293, 15.38400267427140378, 36.05808397467829707 ) ) ;
#24577=CARTESIAN_POINT ( 'NONE',  ( -77.99999999999998579, 42.50000000000000711, 27.50000000000000000 ) ) ;
#24590=CARTESIAN_POINT ( 'NONE',  ( -20.20090942434742587, -32.69829930755841474, 27.50000000000000355 ) ) ;
#24606=AXIS2_PLACEMENT_3D ( 'NONE', #1698, #13866, #10921 ) ;
#24615=CARTESIAN_POINT ( 'NONE',  ( -38.65487109636899277, 5.678429112161928138, 32.12412996058973391 ) ) ;
#24651=CARTESIAN_POINT ( 'NONE',  ( 8.080641794577413606, 38.55540066144438782, 34.49999999999999289 ) ) ;
#24655=CARTESIAN_POINT ( 'NONE',  ( 29.81956388892670873, 15.48018185647901745, 41.40175883629448350 ) ) ;
#24656=ORIENTED_EDGE ( 'NONE', *, *, #7533, .F. ) ;
#24657=CARTESIAN_POINT ( 'NONE',  ( -26.58938213246210580, -6.321715805855834702, 47.66948656093877190 ) ) ;
#24669=CARTESIAN_POINT ( 'NONE',  ( 10.54846567588233697, 41.02342312940356095, 28.96798071624879611 ) ) ;
#24671=CARTESIAN_POINT ( 'NONE',  ( 26.58938213246210580, 6.321715805855839143, 43.42684587381940275 ) ) ;
#24681=CARTESIAN_POINT ( 'NONE',  ( -4.037311857024811879, 39.31355646053943076, 34.49999999999998579 ) ) ;
#24689=DIRECTION ( 'NONE',  ( -0.000000000000000000, -0.000000000000000000, 1.000000000000000000 ) ) ;
#24691=B_SPLINE_CURVE_WITH_KNOTS ( 'NONE', 3,
 ( #7856, #12220, #17050, #361, #19399, #7550 ),
 .UNSPECIFIED., .F., .F.,
 ( 4, 2, 4 ),
 ( 0.003121276445852158229, 0.003498170197137231551, 0.003875063948422304873 ),
 .UNSPECIFIED. ) ;
#24705=CARTESIAN_POINT ( 'NONE',  ( 6.084764702337812636, -42.09022401479442976, 28.87506468199332232 ) ) ;
#24714=CARTESIAN_POINT ( 'NONE',  ( -38.68935852364796801, 5.395939196257416803, 35.04663804086064971 ) ) ;
#24723=ORIENTED_EDGE ( 'NONE', *, *, #42, .F. ) ;
#24745=VECTOR ( 'NONE', #16721, 1000.000000000000000 ) ;
#24767=ADVANCED_FACE ( 'NONE', ( #23171 ), #28445, .T. ) ;
#24768=CARTESIAN_POINT ( 'NONE',  ( -30.63683511483046118, 26.33160370704736408, 30.43224823015176383 ) ) ;
#24791=AXIS2_PLACEMENT_3D ( 'NONE', #18986, #4771, #21770 ) ;
#24837=CARTESIAN_POINT ( 'NONE',  ( 14.93532791487696976, 34.40258920739002235, 37.50000000003241496 ) ) ;
#24849=LINE ( 'NONE', #20160, #14854 ) ;
#24875=CARTESIAN_POINT ( 'NONE',  ( -31.57687401261848592, 15.10620312102103036, 35.75338942089705796 ) ) ;
#24886=CARTESIAN_POINT ( 'NONE',  ( -37.26385291380725562, -4.397137131605170168, 37.49999999999801759 ) ) ;
#24920=APPLICATION_CONTEXT ( 'automotive_design' ) ;
#24927=CARTESIAN_POINT ( 'NONE',  ( 22.11486391166659615, -35.01327975322180919, 29.53756365415747354 ) ) ;
#24957=B_SPLINE_CURVE_WITH_KNOTS ( 'NONE', 3,
 ( #25078, #13086, #22575, #1229 ),
 .UNSPECIFIED., .F., .F.,
 ( 4, 4 ),
 ( 3.022186913382060468E-07, 0.007932103869840195776 ),
 .UNSPECIFIED. ) ;
#24960=B_SPLINE_CURVE_WITH_KNOTS ( 'NONE', 3,
 ( #22860, #3540, #13059, #22549, #25050, #17574, #1201, #6027, #6182, #18041, #1511, #3694, #13208, #27556 ),
 .UNSPECIFIED., .F., .F.,
 ( 4, 2, 2, 2, 2, 2, 4 ),
 ( 2.980251112064282051E-07, 0.0007442722521831252177, 0.001488246479255043997, 0.001860233592791008320, 0.002232220706326972642, 0.002604207819862936965, 0.002976194933398901288 ),
 .UNSPECIFIED. ) ;
#24962=ADVANCED_FACE ( 'NONE', ( #10115 ), #12512, .F. ) ;
#24966=CARTESIAN_POINT ( 'NONE',  ( 0.000000000000000000, 39.50000000000000000, 27.50000000000000355 ) ) ;
#24969=DIRECTION ( 'NONE',  ( -0.000000000000000000, -0.000000000000000000, 1.000000000000000000 ) ) ;
#24987=CYLINDRICAL_SURFACE ( 'NONE', #8990, 1.999999999999998224 ) ;
#25031=CARTESIAN_POINT ( 'NONE',  ( -22.86367660746757480, -34.44063100554308932, 34.50785639329988186 ) ) ;
#25050=CARTESIAN_POINT ( 'NONE',  ( 33.03549465208793379, -8.974030344605372633, 40.76751417242802944 ) ) ;
#25074=DIRECTION ( 'NONE',  ( 0.3598999890241650346, 0.9329908884337541064, 0.000000000000000000 ) ) ;
#25076=EDGE_LOOP ( 'NONE', ( #30317, #4410, #1553, #2812, #23248, #21671 ) ) ;
#25078=CARTESIAN_POINT ( 'NONE',  ( -29.61203839202723032, 15.40012917324033381, 37.38016955275591613 ) ) ;
#25092=CARTESIAN_POINT ( 'NONE',  ( 31.18890335284659443, -19.89223002944918761, 27.50000000000001776 ) ) ;
#25102=CARTESIAN_POINT ( 'NONE',  ( 23.10264100946039534, 11.84391650453516043, 49.03857552305024825 ) ) ;
#25113=ORIENTED_EDGE ( 'NONE', *, *, #18891, .F. ) ;
#25119=CARTESIAN_POINT ( 'NONE',  ( -15.85884089648730644, -35.55173462727348266, 27.49999999999998934 ) ) ;
#25130=CYLINDRICAL_SURFACE ( 'NONE', #27075, 2.000000000000001776 ) ;
#25136=ORIENTED_EDGE ( 'NONE', *, *, #27910, .F. ) ;
#25161=CARTESIAN_POINT ( 'NONE',  ( -33.54113041553378594, 10.01041480049199173, 35.75454235599931252 ) ) ;
#25165=CARTESIAN_POINT ( 'NONE',  ( -29.61203839202723032, 15.40012917324033381, 37.38016955275591613 ) ) ;
#25168=CARTESIAN_POINT ( 'NONE',  ( -5.029589720584652035, -42.14523135961886169, 34.60377126736910469 ) ) ;
#25176=CARTESIAN_POINT ( 'NONE',  ( 0.000000000000000000, 0.000000000000000000, 34.49999999999999289 ) ) ;
#25177=CARTESIAN_POINT ( 'NONE',  ( -9.737156396509783818, -41.16134080394702721, 34.57994222443139165 ) ) ;
#25184=ORIENTED_EDGE ( 'NONE', *, *, #3444, .F. ) ;
#25199=CARTESIAN_POINT ( 'NONE',  ( -32.19782014694307293, 14.25394737442115733, 39.78814634291943975 ) ) ;
#25221=CARTESIAN_POINT ( 'NONE',  ( -8.549354426873712498, 36.53117268482988322, 37.50000000000129319 ) ) ;
#25225=CARTESIAN_POINT ( 'NONE',  ( 32.28307784207223108, -8.475829241206289666, 41.62281023987511475 ) ) ;
#25227=AXIS2_PLACEMENT_3D ( 'NONE', #24425, #22080, #21466 ) ;
#25232=CARTESIAN_POINT ( 'NONE',  ( 24.12434750488276691, -33.40019891058758361, 29.69951012705165283 ) ) ;
#25242=VECTOR ( 'NONE', #20055, 1000.000000000000000 ) ;
#25243=CARTESIAN_POINT ( 'NONE',  ( 9.268856789657281325, -38.25380398711768493, 27.49999999999999645 ) ) ;
#25258=DIRECTION ( 'NONE',  ( 1.000000000000000000, 0.000000000000000000, 0.000000000000000000 ) ) ;
#25276=CARTESIAN_POINT ( 'NONE',  ( -4.375757216953428294E-15, -39.50000000000000000, 34.80090346875804386 ) ) ;
#25300=CARTESIAN_POINT ( 'NONE',  ( -33.43088607478084384, -9.613432587296607323, 35.97188228570009727 ) ) ;
#25319=B_SPLINE_CURVE_WITH_KNOTS ( 'NONE', 3,
 ( #14336, #2492, #23389, #26356 ),
 .UNSPECIFIED., .F., .F.,
 ( 4, 4 ),
 ( 2.143643656977389965E-07, 0.003421830178490238485 ),
 .UNSPECIFIED. ) ;
#25327=CARTESIAN_POINT ( 'NONE',  ( -32.49060333908415288, 8.555881924488323520, 37.15911814905553001 ) ) ;
#25333=CARTESIAN_POINT ( 'NONE',  ( 19.81438245631380113, -36.63624637273056095, 34.51461286089641334 ) ) ;
#25343=CARTESIAN_POINT ( 'NONE',  ( -10.60011131210715440, -35.97541730661800585, 37.50000000000953548 ) ) ;
#25344=EDGE_CURVE ( 'NONE', #27501, #19329, #8827, .T. ) ;
#25345=ORIENTED_EDGE ( 'NONE', *, *, #24384, .T. ) ;
#25386=CARTESIAN_POINT ( 'NONE',  ( -0.4404457618616001158, 37.56938067690362715, 37.49999999996049382 ) ) ;
#25409=CARTESIAN_POINT ( 'NONE',  ( 28.55068628633582861, -24.19494186940697844, 27.50000000000000355 ) ) ;
#25414=PLANE ( 'NONE',  #9322 ) ;
#25419=CARTESIAN_POINT ( 'NONE',  ( 23.59223810913926656, 12.86535672232149707, 48.12792051025102325 ) ) ;
#25423=CARTESIAN_POINT ( 'NONE',  ( -33.19297012087366028, -9.154531925606914200, 40.56825029428927110 ) ) ;
#25438=CARTESIAN_POINT ( 'NONE',  ( -34.83396020575242602, 10.30249279383516381, 34.80090346875805096 ) ) ;
#25455=CARTESIAN_POINT ( 'NONE',  ( -7.946654084575756727, 38.53100927994441349, 27.50000000000000711 ) ) ;
#25457=CARTESIAN_POINT ( 'NONE',  ( 23.15419545472249041, -10.94206393902796925, 49.39104690845173451 ) ) ;
#25493=CARTESIAN_POINT ( 'NONE',  ( 37.99594503683577074, -9.942093294496530120, 34.97541777410600616 ) ) ;
#25501=EDGE_CURVE ( 'NONE', #11387, #26848, #10015, .T. ) ;
#25504=CARTESIAN_POINT ( 'NONE',  ( -15.50214450999369831, -39.10813156751746789, 34.54020706897479442 ) ) ;
#25506=CARTESIAN_POINT ( 'NONE',  ( -27.03074382657074537, -6.449748410230988327, 42.96778633356042576 ) ) ;
#25540=B_SPLINE_CURVE_WITH_KNOTS ( 'NONE', 3,
 ( #490, #17643, #27160, #26690, #5786, #7818, #17329, #24344, #29346, #2991, #7988, #17490, #12510, #27012, #5640, #15135, #14830, #956, #22312, #10467, #5319, #12665, #24651, #3286, #19516, #24497, #22004, #14983 ),
 .UNSPECIFIED., .F., .F.,
 ( 4, 2, 2, 2, 2, 2, 2, 2, 2, 2, 2, 2, 2, 4 ),
 ( 0.06961508940978108906, 0.07265001228952157331, 0.07416747372939182237, 0.07568493516926205755, 0.08175478092874302605, 0.08782462668822399454, 0.09085954956796447879, 0.09389447244770496304, 0.09996431820718593153, 0.1029992410869264019, 0.1060341639666669000, 0.1121040097261478685, 0.1151389326058883389, 0.1181738554856288231 ),
 .UNSPECIFIED. ) ;
#25548=CARTESIAN_POINT ( 'NONE',  ( 24.75800239156184190, -7.045788922043113800, 49.25937209215325652 ) ) ;
#25552=ORIENTED_EDGE ( 'NONE', *, *, #3444, .T. ) ;
#25553=CARTESIAN_POINT ( 'NONE',  ( 35.76481447503398670, -5.202797454133663457, 27.50000000000001066 ) ) ;
#25576=CARTESIAN_POINT ( 'NONE',  ( 33.42925964089141644, -11.06161099612213228, -16.55003854064094426 ) ) ;
#25586=CARTESIAN_POINT ( 'NONE',  ( -35.76481447503397959, 5.202797454133647470, 34.80090346875805096 ) ) ;
#25606=CARTESIAN_POINT ( 'NONE',  ( -26.85023221529805681, 26.31525925951064337, 27.50000000000000355 ) ) ;
#25608=DIRECTION ( 'NONE',  ( -1.000000000000000000, 0.000000000000000000, 0.000000000000000000 ) ) ;
#25613=DIRECTION ( 'NONE',  ( -0.000000000000000000, -0.000000000000000000, -1.000000000000000000 ) ) ;
#25643=CARTESIAN_POINT ( 'NONE',  ( 10.21997447646774937, -36.08534693423421658, 37.50000000003055334 ) ) ;
#25644=CYLINDRICAL_SURFACE ( 'NONE', #7609, 22.49999999999996447 ) ;
#25650=ORIENTED_EDGE ( 'NONE', *, *, #19093, .T. ) ;
#25653=CARTESIAN_POINT ( 'NONE',  ( -25.18096005886327760, -6.640581704039635547, 44.71664046397099668 ) ) ;
#25658=CARTESIAN_POINT ( 'NONE',  ( -24.35970437652574105, 13.37404834226503247, 47.21042702067971675 ) ) ;
#25671=ORIENTED_EDGE ( 'NONE', *, *, #16974, .T. ) ;
#25680=EDGE_LOOP ( 'NONE', ( #11911, #4660, #22503, #10062, #5124 ) ) ;
#25686=DIRECTION ( 'NONE',  ( -0.9329908884337534403, 0.3598999890241668664, 0.000000000000000000 ) ) ;
#25695=EDGE_CURVE ( 'NONE', #29313, #1784, #15558, .T. ) ;
#25696=VECTOR ( 'NONE', #5367, 1000.000000000000000 ) ;
#25703=CARTESIAN_POINT ( 'NONE',  ( 36.00000000000001421, 2.601438916704194249, 34.80090346875809360 ) ) ;
#25710=FACE_OUTER_BOUND ( 'NONE', #10707, .T. ) ;
#25711=DIRECTION ( 'NONE',  ( -1.000000000000000000, 0.000000000000000000, 0.000000000000000000 ) ) ;
#25715=DIRECTION ( 'NONE',  ( -0.000000000000000000, -0.000000000000000000, 1.000000000000000000 ) ) ;
#25722=ORIENTED_EDGE ( 'NONE', *, *, #12282, .F. ) ;
#25728=ADVANCED_FACE ( 'NONE', ( #10891 ), #26854, .F. ) ;
#25729=CARTESIAN_POINT ( 'NONE',  ( -34.83396020575241891, -10.30249279383514960, 27.50000000000001066 ) ) ;
#25745=CARTESIAN_POINT ( 'NONE',  ( 36.00000000000063238, 1.782879839924971010, 34.75735931288080849 ) ) ;
#25749=CARTESIAN_POINT ( 'NONE',  ( 23.59634279088906439, -12.86962927293162906, 48.12226976371609766 ) ) ;
#25755=CARTESIAN_POINT ( 'NONE',  ( 30.53339558441486190, 7.800891647352844238, 43.48653168448679196 ) ) ;
#25763=CARTESIAN_POINT ( 'NONE',  ( 21.15904228388716746, -31.96044797056314124, 27.50000000000000355 ) ) ;
#25775=ORIENTED_EDGE ( 'NONE', *, *, #25807, .T. ) ;
#25788=CARTESIAN_POINT ( 'NONE',  ( 33.42925964089141644, 11.06161099612213405, -16.55003854064094426 ) ) ;
#25794=CARTESIAN_POINT ( 'NONE',  ( 26.15871596101562702, -26.98401179872733735, 37.49999999983522514 ) ) ;
#25802=ORIENTED_EDGE ( 'NONE', *, *, #42, .T. ) ;
#25803=DIRECTION ( 'NONE',  ( 1.000000000000000000, 0.000000000000000000, 0.000000000000000000 ) ) ;
#25805=CARTESIAN_POINT ( 'NONE',  ( -30.50204315964898427, -15.53056155674291183, 40.77182279853386859 ) ) ;
#25807=EDGE_CURVE ( 'NONE', #28109, #28104, #17458, .T. ) ;
#25810=CARTESIAN_POINT ( 'NONE',  ( 29.81954908927654202, -15.48017614753372584, 41.40177460054268721 ) ) ;
#25829=LINE ( 'NONE', #11334, #27418 ) ;
#25846=CARTESIAN_POINT ( 'NONE',  ( -37.63189979596968016, 11.23836474745404423, 34.94552664686906951 ) ) ;
#25855=FACE_OUTER_BOUND ( 'NONE', #28841, .T. ) ;
#25864=CARTESIAN_POINT ( 'NONE',  ( 4.677126025380971441, 39.24912351428226742, 27.50000000000000355 ) ) ;
#25870=CYLINDRICAL_SURFACE ( 'NONE', #12171, 2.000000000000001776 ) ;
#25881=AXIS2_PLACEMENT_3D ( 'NONE', #6392, #6230, #25711 ) ;
#25883=FACE_BOUND ( 'NONE', #14801, .T. ) ;
#25891=CARTESIAN_POINT ( 'NONE',  ( 8.029152834601454458, -38.52032120320185271, 34.49999999999999289 ) ) ;
#25898=CARTESIAN_POINT ( 'NONE',  ( -23.07950435457351190, 11.50806656539842798, 44.96784366550151191 ) ) ;
#25902=ORIENTED_EDGE ( 'NONE', *, *, #22130, .T. ) ;
#25915=CARTESIAN_POINT ( 'NONE',  ( 21.62415194650660766, 31.60332031111338225, 27.50000000000000000 ) ) ;
#25932=EDGE_CURVE ( 'NONE', #30628, #165, #6292, .T. ) ;
#25936=LINE ( 'NONE', #28290, #19618 ) ;
#25938=CARTESIAN_POINT ( 'NONE',  ( 10.78888246121507599, -35.91932794629070003, 37.50000000001028866 ) ) ;
#25939=ADVANCED_FACE ( 'NONE', ( #8858 ), #20689, .F. ) ;
#25974=CARTESIAN_POINT ( 'NONE',  ( 32.60608336680204644, -8.625548295239457985, 37.02973996997542372 ) ) ;
#25977=CARTESIAN_POINT ( 'NONE',  ( 37.49999999999997158, 1.387778780781445676E-14, 37.50000000000000000 ) ) ;
#25995=CARTESIAN_POINT ( 'NONE',  ( -27.00603848422143471, 26.04669493682374437, 37.49999999997637445 ) ) ;
#25999=CARTESIAN_POINT ( 'NONE',  ( 32.28307784207223108, 8.475829241206289666, 37.38016955275583086 ) ) ;
#26004=CARTESIAN_POINT ( 'NONE',  ( 27.03074382657074182, -6.449748410230990991, 42.96778633356034049 ) ) ;
#26008=CARTESIAN_POINT ( 'NONE',  ( 25.18466322232234234, -6.657711795334220639, 48.95036236631847260 ) ) ;
#26013=EDGE_CURVE ( 'NONE', #19602, #10953, #30450, .T. ) ;
#26018=ORIENTED_EDGE ( 'NONE', *, *, #9763, .T. ) ;
#26026=CARTESIAN_POINT ( 'NONE',  ( -25.53015708495999903, 6.470147010658195974, 48.66282223834838305 ) ) ;
#26035=CARTESIAN_POINT ( 'NONE',  ( -6.397449029611151694, -41.94755430240511629, 28.88750951715501714 ) ) ;
#26066=CARTESIAN_POINT ( 'NONE',  ( 29.09438610025163641, 23.39414391798310078, 27.50000000000000355 ) ) ;
#26088=CARTESIAN_POINT ( 'NONE',  ( 29.37505062631091945, 27.96840008810541178, 34.56100623550605633 ) ) ;
#26118=CARTESIAN_POINT ( 'NONE',  ( 6.601643239663004076E-16, 42.50000000000000000, 28.83974596215562514 ) ) ;
#26136=CARTESIAN_POINT ( 'NONE',  ( -27.78122617307444031, 29.83607645924699270, 30.06620328777349016 ) ) ;
#26138=CARTESIAN_POINT ( 'NONE',  ( 23.21352257770656635, -10.78826658734920052, -16.55003854064094426 ) ) ;
#26152=CYLINDRICAL_SURFACE ( 'NONE', #25227, 1.999999999999998224 ) ;
#26180=ADVANCED_FACE ( 'NONE', ( #8200 ), #27224, .F. ) ;
#26198=DIRECTION ( 'NONE',  ( 0.3598999890241665334, -0.9329908884337535513, 0.000000000000000000 ) ) ;
#26202=CARTESIAN_POINT ( 'NONE',  ( -18.68130254075365215, -33.76891359627503419, 27.50000000000000711 ) ) ;
#26205=CARTESIAN_POINT ( 'NONE',  ( -25.25456494851459865, -28.22455358388291202, 34.49999999999998579 ) ) ;
#26216=CARTESIAN_POINT ( 'NONE',  ( 2.477745044295800891, 39.41216975536991640, 27.50000000000000000 ) ) ;
#26220=AXIS2_PLACEMENT_3D ( 'NONE', #10985, #18155, #20486 ) ;
#26239=CARTESIAN_POINT ( 'NONE',  ( 36.99855377474076334, 13.50962263858970225, 34.89305612718171545 ) ) ;
#26284=ORIENTED_EDGE ( 'NONE', *, *, #15464, .F. ) ;
#26291=AXIS2_PLACEMENT_3D ( 'NONE', #9826, #26198, #303 ) ;
#26295=CARTESIAN_POINT ( 'NONE',  ( -38.30462971311529685, 8.019294621567119918, 35.00802478783429450 ) ) ;
#26300=CARTESIAN_POINT ( 'NONE',  ( 33.26833594138172145, 9.291422874672347731, 36.21597341152490657 ) ) ;
#26301=PLANE ( 'NONE',  #24791 ) ;
#26303=VERTEX_POINT ( 'NONE', #14413 ) ;
#26309=CARTESIAN_POINT ( 'NONE',  ( -4.776122516674677878E-15, -42.50000000000000000, 27.50000000000000355 ) ) ;
#26321=ORIENTED_EDGE ( 'NONE', *, *, #16974, .F. ) ;
#26337=EDGE_CURVE ( 'NONE', #5196, #5082, #17552, .T. ) ;
#26345=CARTESIAN_POINT ( 'NONE',  ( 30.17204898946756586, 26.93709580362141409, 30.36897652752471188 ) ) ;
#26356=CARTESIAN_POINT ( 'NONE',  ( 24.44496207165490631, -7.595930209050163029, 45.15942333309103418 ) ) ;
#26366=CARTESIAN_POINT ( 'NONE',  ( -29.06589025085023081, -23.33669524104240978, 27.50000000000000711 ) ) ;
#26370=ADVANCED_FACE ( 'NONE', ( #24214 ), #5512, .F. ) ;
#26373=CARTESIAN_POINT ( 'NONE',  ( -36.00000000000000000, -1.100768691257133318E-12, 34.75735931288076586 ) ) ;
#26393=ORIENTED_EDGE ( 'NONE', *, *, #7533, .T. ) ;
#26409=CARTESIAN_POINT ( 'NONE',  ( 21.70146777712312769, 30.67724188593774670, 37.49999999988722266 ) ) ;
#26413=CARTESIAN_POINT ( 'NONE',  ( -23.12263228470263243, -11.97179573940914921, 44.71970589514035765 ) ) ;
#26442=( BOUNDED_CURVE ( )  B_SPLINE_CURVE ( 3, ( #16794, #14754, #14611, #26309 ),
 .UNSPECIFIED., .F., .T. ) 
 B_SPLINE_CURVE_WITH_KNOTS ( ( 4, 4 ),
 ( 0.000000000000000000, 3.141592653589793116 ),
 .UNSPECIFIED. ) 
 CURVE ( )  GEOMETRIC_REPRESENTATION_ITEM ( )  RATIONAL_B_SPLINE_CURVE ( ( 1.000000000000000000, 0.3333333333333333703, 0.3333333333333333703, 1.000000000000000000 ) ) 
 REPRESENTATION_ITEM ( '' )  );
#26454=DIRECTION ( 'NONE',  ( 0.3598999890241654231, 0.9329908884337539954, 0.000000000000000000 ) ) ;
#26456=CARTESIAN_POINT ( 'NONE',  ( -36.51119354604474410, 15.00142784232802740, 34.85629366384495853 ) ) ;
#26471=ORIENTED_EDGE ( 'NONE', *, *, #2163, .F. ) ;
#26472=CARTESIAN_POINT ( 'NONE',  ( -26.31094384852241319, 8.315730187098489878, -16.55003854064094426 ) ) ;
#26473=CARTESIAN_POINT ( 'NONE',  ( 2.338573377552017440, 39.50000000000000711, 34.80090346875810781 ) ) ;
#26475=ORIENTED_EDGE ( 'NONE', *, *, #19093, .F. ) ;
#26478=B_SPLINE_CURVE_WITH_KNOTS ( 'NONE', 3,
 ( #23096, #28101, #6722, #16234, #17154, #7800, #26523, #26373 ),
 .UNSPECIFIED., .F., .F.,
 ( 4, 2, 2, 4 ),
 ( 0.000000000000000000, 0.005288043134231363955, 0.007932064701347045499, 0.01057608626846272791 ),
 .UNSPECIFIED. ) ;
#26481=VECTOR ( 'NONE', #18038, 1000.000000000000000 ) ;
#26489=CARTESIAN_POINT ( 'NONE',  ( 23.59634279088906439, -12.86962927293163084, 43.87962907659681377 ) ) ;
#26493=CARTESIAN_POINT ( 'NONE',  ( 18.35592613994001709, 37.52326638810179560, 29.29232531120126737 ) ) ;
#26506=DIRECTION ( 'NONE',  ( -0.000000000000000000, -0.000000000000000000, 1.000000000000000000 ) ) ;
#26523=CARTESIAN_POINT ( 'NONE',  ( -36.00000000000002842, 0.8865895960648689789, 34.75735931288077296 ) ) ;
#26550=EDGE_CURVE ( 'NONE', #14452, #17402, #21068, .T. ) ;
#26553=CYLINDRICAL_SURFACE ( 'NONE', #29674, 1.999999999999998224 ) ;
#26561=CARTESIAN_POINT ( 'NONE',  ( 34.26660261194440693, 20.46295234328604096, 31.03790124022056318 ) ) ;
#26574=VERTEX_POINT ( 'NONE', #28262 ) ;
#26579=CARTESIAN_POINT ( 'NONE',  ( -32.02118151871192708, 18.16475142757035144, 34.49999999999999289 ) ) ;
#26580=AXIS2_PLACEMENT_3D ( 'NONE', #13768, #29860, #13484 ) ;
#26583=CIRCLE ( 'NONE', #673, 37.50000000000001421 ) ;
#26596=CARTESIAN_POINT ( 'NONE',  ( -23.36055057548231417, 12.54866584153426423, 44.23986152793528248 ) ) ;
#26615=CARTESIAN_POINT ( 'NONE',  ( -36.33684937716974872, -15.65606802492079730, 31.48606577064049006 ) ) ;
#26619=CARTESIAN_POINT ( 'NONE',  ( 33.56327786402390245, 10.34181101807379299, 35.63689980405264635 ) ) ;
#26633=DIRECTION ( 'NONE',  ( -0.000000000000000000, -0.000000000000000000, 1.000000000000000000 ) ) ;
#26634=ORIENTED_EDGE ( 'NONE', *, *, #20420, .F. ) ;
#26650=CARTESIAN_POINT ( 'NONE',  ( 17.21962637186833334, 38.15825840448668771, 29.23201136369613451 ) ) ;
#26655=CARTESIAN_POINT ( 'NONE',  ( -38.85201932933775026, 3.754465866770057225, 32.18529919512457127 ) ) ;
#26672=CARTESIAN_POINT ( 'NONE',  ( -20.76850923836823526, -32.27873595568063081, 34.50000000000000000 ) ) ;
#26690=CARTESIAN_POINT ( 'NONE',  ( 33.70141996666045259, 13.89393473031433324, 34.49999999999999289 ) ) ;
#26691=CARTESIAN_POINT ( 'NONE',  ( -36.00000000000000000, -1.100768691257133318E-12, 34.75735931288076586 ) ) ;
#26709=CARTESIAN_POINT ( 'NONE',  ( 39.00460276462784748, -0.1210056128972753636, 35.08014749300483004 ) ) ;
#26724=CARTESIAN_POINT ( 'NONE',  ( -30.53339558441486190, -7.800891647352837133, 43.48653168448686301 ) ) ;
#26732=EDGE_CURVE ( 'NONE', #13217, #11117, #17166, .T. ) ;
#26738=EDGE_CURVE ( 'NONE', #3711, #17402, #21168, .T. ) ;
#26744=DIRECTION ( 'NONE',  ( -0.000000000000000000, -0.000000000000000000, -1.000000000000000000 ) ) ;
#26746=CARTESIAN_POINT ( 'NONE',  ( -23.21352257770656990, -10.78826658734919519, 49.40206402021038201 ) ) ;
#26771=CARTESIAN_POINT ( 'NONE',  ( -39.07105923661990943, -0.5277388387263558522, 35.08714678962015654 ) ) ;
#26772=ORIENTED_EDGE ( 'NONE', *, *, #29197, .T. ) ;
#26783=CLOSED_SHELL ( 'NONE', ( #24767, #11304, #17210, #8236, #4971, #22973, #10301, #29596, #8047, #27095, #24962, #1733, #14511, #13770, #23296, #19470, #30315, #5965, #27149, #22346, #16672, #28069, #6843, #14471, #28604, #24134, #27503, #22186, #16287, #3875, #26180, #691, #11089, #15722, #25939, #4997, #4500, #4194, #25728, #17982, #9586, #15084, #4600, #15893, #21377, #23294, #17030, #10229, #8438, #23885, #11260, #26370, #19633, #22891 ) ) ;
#26814=CARTESIAN_POINT ( 'NONE',  ( 23.20389136007291953, -12.24563090271730736, 44.52079389607786197 ) ) ;
#26815=CARTESIAN_POINT ( 'NONE',  ( 1.236805935716845939, 39.48255573641029770, 27.50000000000001066 ) ) ;
#26819=CARTESIAN_POINT ( 'NONE',  ( -3.696774448978239480, -32.23395975793253854, 28.87158698979378002 ) ) ;
#26825=CARTESIAN_POINT ( 'NONE',  ( -38.37115330322435369, -7.710785714854020867, 32.03772168544337262 ) ) ;
#26843=CARTESIAN_POINT ( 'NONE',  ( -31.12530087898743503, -19.95159923194576379, 34.50000000000000000 ) ) ;
#26848=VERTEX_POINT ( 'NONE', #10150 ) ;
#26850=EDGE_LOOP ( 'NONE', ( #26471, #17446, #13388, #11580, #13907 ) ) ;
#26854=PLANE ( 'NONE',  #15520 ) ;
#26861=CARTESIAN_POINT ( 'NONE',  ( -4.677126025380957230, 39.24912351428227453, 27.50000000000000355 ) ) ;
#26876=CARTESIAN_POINT ( 'NONE',  ( 15.64865523245225631, 38.95674053321715746, 29.15699439579599783 ) ) ;
#26883=CARTESIAN_POINT ( 'NONE',  ( -23.26222494989736234, -12.36939612486375495, 44.41134540914034545 ) ) ;
#26888=PRODUCT ( 'Vane Snap Cap', 'Vane Snap Cap', '', ( #3047 ) ) ;
#26891=CARTESIAN_POINT ( 'NONE',  ( -20.72875052343767521, 32.30954557037109964, 34.49999999999999289 ) ) ;
#26910=ORIENTED_EDGE ( 'NONE', *, *, #807, .F. ) ;
#26914=CARTESIAN_POINT ( 'NONE',  ( -3.112355512349863851, -37.38886688928499069, 37.50000000001043787 ) ) ;
#26928=CARTESIAN_POINT ( 'NONE',  ( -37.08962926481365940, -5.682944862436646538, 37.49999999998664890 ) ) ;
#26932=CARTESIAN_POINT ( 'NONE',  ( 27.03074382657074537, -6.449748410230991880, -16.55003854064094426 ) ) ;
#26937=CARTESIAN_POINT ( 'NONE',  ( 32.06725342158288328, 14.54034564589948708, 35.54788606881758994 ) ) ;
#26944=CARTESIAN_POINT ( 'NONE',  ( 0.000000000000000000, 42.50000000000000000, 27.50000000000000355 ) ) ;
#26946=EDGE_CURVE ( 'NONE', #22873, #20218, #10824, .T. ) ;
#26957=CARTESIAN_POINT ( 'NONE',  ( -35.93563768862540542, 2.440659245201815430, 27.50000000000000355 ) ) ;
#26963=CARTESIAN_POINT ( 'NONE',  ( -27.03074382657074182, -6.449748410230987439, 47.21042702067970964 ) ) ;
#26973=CARTESIAN_POINT ( 'NONE',  ( 38.94223652925970924, 2.647167246129292550, 32.21377772506992443 ) ) ;
#26978=CARTESIAN_POINT ( 'NONE',  ( -16.13886355804662998, 38.71476141167133278, 29.17969182664677419 ) ) ;
#26983=CARTESIAN_POINT ( 'NONE',  ( 34.70577939417261604, -10.49309206032036634, 34.49999999999999289 ) ) ;
#27007=CARTESIAN_POINT ( 'NONE',  ( -25.41307773079512344, 6.523700759042258213, 44.52046879171667371 ) ) ;
#27012=CARTESIAN_POINT ( 'NONE',  ( 23.79391290694626093, 29.65739006622967011, 34.50000000000000711 ) ) ;
#27013=CARTESIAN_POINT ( 'NONE',  ( -23.69412710310941961, 29.84645176427129698, 34.80090346875805096 ) ) ;
#27019=CARTESIAN_POINT ( 'NONE',  ( 23.21352257770656635, -10.78826658734920052, 49.40206402021031806 ) ) ;
#27024=AXIS2_PLACEMENT_3D ( 'NONE', #7858, #672, #15015 ) ;
#27027=CARTESIAN_POINT ( 'NONE',  ( 17.48232412878148878, 37.99796894973091099, 29.24739480102024558 ) ) ;
#27030=CARTESIAN_POINT ( 'NONE',  ( -33.56595177138117947, -10.45696648424866204, 35.60059606545802779 ) ) ;
#27053=CIRCLE ( 'NONE', #20560, 10.00000000000000000 ) ;
#27059=ORIENTED_EDGE ( 'NONE', *, *, #1210, .T. ) ;
#27060=CARTESIAN_POINT ( 'NONE',  ( 5.060094141397912360, 42.14075867279367316, 28.87075318537527835 ) ) ;
#27062=CARTESIAN_POINT ( 'NONE',  ( 2.598297338551552205, -42.41243084101535032, 28.84727347638572681 ) ) ;
#27071=CARTESIAN_POINT ( 'NONE',  ( -32.99004629359474450, -22.67711567301405395, 30.80987819614264112 ) ) ;
#27075=AXIS2_PLACEMENT_3D ( 'NONE', #3773, #13293, #22788 ) ;
#27095=ADVANCED_FACE ( 'NONE', ( #9048, #25883, #11543 ), #6608, .T. ) ;
#27101=CARTESIAN_POINT ( 'NONE',  ( -35.73758792595601363, 4.918610258824734238, 27.49999999999999645 ) ) ;
#27119=CARTESIAN_POINT ( 'NONE',  ( 13.78074022358099704, -39.76440514451509500, 29.08269373213634168 ) ) ;
#27124=CARTESIAN_POINT ( 'NONE',  ( -23.10040941844921392, -34.24922087329859721, 29.61388150951794884 ) ) ;
#27133=ORIENTED_EDGE ( 'NONE', *, *, #26732, .T. ) ;
#27134=CARTESIAN_POINT ( 'NONE',  ( 33.42925964089140933, 11.06161099612213405, 35.54550565580007060 ) ) ;
#27147=ORIENTED_EDGE ( 'NONE', *, *, #17633, .F. ) ;
#27149=ADVANCED_FACE ( 'NONE', ( #14167 ), #2172, .F. ) ;
#27160=CARTESIAN_POINT ( 'NONE',  ( 34.17801210021485758, 12.44599808121550844, 34.49999999999999289 ) ) ;
#27165=ORIENTED_EDGE ( 'NONE', *, *, #18176, .T. ) ;
#27169=CARTESIAN_POINT ( 'NONE',  ( -23.07950435457351190, 11.50806656539842798, 44.96784366550151191 ) ) ;
#27178=EDGE_CURVE ( 'NONE', #4181, #27891, #27053, .T. ) ;
#27185=ORIENTED_EDGE ( 'NONE', *, *, #21704, .F. ) ;
#27194=CARTESIAN_POINT ( 'NONE',  ( -27.03074382657074537, 6.449748410230984774, 42.96778633356043287 ) ) ;
#27196=DIRECTION ( 'NONE',  ( 0.3598999890241647570, -0.9329908884337542174, 0.000000000000000000 ) ) ;
#27197=CARTESIAN_POINT ( 'NONE',  ( -32.19782014694307293, -14.25394737442115733, -16.55003854064094426 ) ) ;
#27199=ORIENTED_EDGE ( 'NONE', *, *, #12678, .F. ) ;
#27214=AXIS2_PLACEMENT_3D ( 'NONE', #8247, #12937, #1233 ) ;
#27219=CARTESIAN_POINT ( 'NONE',  ( -25.72578587384908388, -31.97238736827291561, 29.84495957342102201 ) ) ;
#27220=ORIENTED_EDGE ( 'NONE', *, *, #18006, .F. ) ;
#27224=PLANE ( 'NONE',  #24510 ) ;
#27230=CARTESIAN_POINT ( 'NONE',  ( 30.74147208807243103, 15.49548351932574519, 36.33144972441040466 ) ) ;
#27262=ORIENTED_EDGE ( 'NONE', *, *, #12035, .T. ) ;
#27270=CARTESIAN_POINT ( 'NONE',  ( 35.81403885549343613, -16.83674392041570655, 31.37468618001539156 ) ) ;
#27284=VERTEX_POINT ( 'NONE', #14638 ) ;
#27298=EDGE_CURVE ( 'NONE', #12912, #17814, #29768, .T. ) ;
#27308=CARTESIAN_POINT ( 'NONE',  ( 31.10500197267672817, -15.38309308716404900, 36.05646065676224765 ) ) ;
#27313=EDGE_CURVE ( 'NONE', #19828, #7486, #24957, .T. ) ;
#27319=DIRECTION ( 'NONE',  ( 1.000000000000000000, 0.000000000000000000, 0.000000000000000000 ) ) ;
#27342=CARTESIAN_POINT ( 'NONE',  ( -33.42925964089141644, -11.06161099612212695, -16.55003854064094426 ) ) ;
#27346=CARTESIAN_POINT ( 'NONE',  ( -33.25379661643704310, 9.265521131796550236, 40.47962024272059267 ) ) ;
#27375=CARTESIAN_POINT ( 'NONE',  ( -32.94612346989018192, 8.892333671926630601, 36.63232123319113498 ) ) ;
#27389=CARTESIAN_POINT ( 'NONE',  ( -6.588341431580430729, -36.93554111252256433, 37.49999999995496580 ) ) ;
#27408=CARTESIAN_POINT ( 'NONE',  ( 36.00000000000000000, -1.546978760965586295E-11, 34.75735931288068059 ) ) ;
#27412=EDGE_LOOP ( 'NONE', ( #30441, #6808, #27768, #16510 ) ) ;
#27418=VECTOR ( 'NONE', #4462, 1000.000000000000000 ) ;
#27426=CARTESIAN_POINT ( 'NONE',  ( -8.848822535149219348, 41.41987577336931992, 28.93372982618284794 ) ) ;
#27444=EDGE_LOOP ( 'NONE', ( #9318, #25802, #21649, #27199 ) ) ;
#27470=CARTESIAN_POINT ( 'NONE',  ( -23.69412710310941605, -29.84645176427128987, 27.50000000000000355 ) ) ;
#27479=ORIENTED_EDGE ( 'NONE', *, *, #30170, .F. ) ;
#27495=CARTESIAN_POINT ( 'NONE',  ( -33.43024933835881285, 9.611735609129382851, 40.21560466195906258 ) ) ;
#27501=VERTEX_POINT ( 'NONE', #8024 ) ;
#27503=ADVANCED_FACE ( 'NONE', ( #1144 ), #17677, .F. ) ;
#27522=CARTESIAN_POINT ( 'NONE',  ( -33.37677408195396112, 9.488883682882484294, 36.05808397461573378 ) ) ;
#27523=ORIENTED_EDGE ( 'NONE', *, *, #14389, .T. ) ;
#27527=CARTESIAN_POINT ( 'NONE',  ( -1.946983950544124875, -37.46784418063916178, 37.49999999996633449 ) ) ;
#27538=CARTESIAN_POINT ( 'NONE',  ( -18.19086450879680683, -37.70413644374980322, 29.27365136405585488 ) ) ;
#27544=CARTESIAN_POINT ( 'NONE',  ( 23.15418787629628739, 10.94208358504856804, 45.14840481401043348 ) ) ;
#27547=CARTESIAN_POINT ( 'NONE',  ( 30.86161751192251756, 15.46691422980912911, 36.23697955569760865 ) ) ;
#27556=CARTESIAN_POINT ( 'NONE',  ( 33.56327786402390245, -10.34181101807379477, 39.87954049117192312 ) ) ;
#27574=CARTESIAN_POINT ( 'NONE',  ( -15.69812257003878742, 38.91317198416786738, 34.53890312238223714 ) ) ;
#27583=CARTESIAN_POINT ( 'NONE',  ( 36.48404635224623149, -15.03172480188603899, 31.53210484354143617 ) ) ;
#27594=B_SPLINE_CURVE_WITH_KNOTS ( 'NONE', 3,
 ( #24369, #3013, #26413, #26883, #17355, #5503, #28750, #29370, #12209, #19684 ),
 .UNSPECIFIED., .F., .F.,
 ( 4, 2, 2, 2, 4 ),
 ( 0.0007598054600062436074, 0.001542965791078104807, 0.002326126122149965898, 0.003109286453221827423, 0.003892446784293688514 ),
 .UNSPECIFIED. ) ;
#27597=CARTESIAN_POINT ( 'NONE',  ( 21.86019681245147339, 31.48592878035296749, 27.50000000000001066 ) ) ;
#27606=CARTESIAN_POINT ( 'NONE',  ( -28.78283879316666471, 7.125616703334841873, 45.34931131770228063 ) ) ;
#27622=CARTESIAN_POINT ( 'NONE',  ( -2.338573377552017440, -39.49999999999999289, 34.80090346875804386 ) ) ;
#27639=CARTESIAN_POINT ( 'NONE',  ( -22.62322288457161790, 30.83399541182840409, 27.50000000000000711 ) ) ;
#27642=CARTESIAN_POINT ( 'NONE',  ( -32.49058853941425440, -8.555876215535434426, 37.15913391332472315 ) ) ;
#27645=ORIENTED_EDGE ( 'NONE', *, *, #29590, .T. ) ;
#27669=VECTOR ( 'NONE', #7542, 1000.000000000000000 ) ;
#27672=CARTESIAN_POINT ( 'NONE',  ( 17.49967083908764565, -38.01026090106176980, 34.52681008576058019 ) ) ;
#27681=CARTESIAN_POINT ( 'NONE',  ( -23.26222494989734813, -12.36939612486375495, 48.65398609625962933 ) ) ;
#27682=STYLED_ITEM('',(#30886),#3432);
#27686=CARTESIAN_POINT ( 'NONE',  ( -26.58938213246210580, -6.321715805855834702, 43.42684587381948091 ) ) ;
#27711=LINE ( 'NONE', #9136, #30816 ) ;
#27722=CARTESIAN_POINT ( 'NONE',  ( -31.46019086465472725, -15.19107625323260180, 35.82171084658602211 ) ) ;
#27725=CARTESIAN_POINT ( 'NONE',  ( 5.060094141397912360, 42.14075867279367316, 28.87075318537528190 ) ) ;
#27730=CARTESIAN_POINT ( 'NONE',  ( -26.12047388987420149, 6.311255530320346807, 43.88527982295141783 ) ) ;
#27737=CARTESIAN_POINT ( 'NONE',  ( 36.04561543331149664, -16.23932455912026640, 31.42798667167778248 ) ) ;
#27738=DIRECTION ( 'NONE',  ( -0.000000000000000000, -0.000000000000000000, 1.000000000000000000 ) ) ;
#27747=EDGE_CURVE ( 'NONE', #2953, #27284, #30092, .T. ) ;
#27750=CARTESIAN_POINT ( 'NONE',  ( 23.69412710310940540, -29.84645176427128987, 27.50000000000000355 ) ) ;
#27753=FACE_OUTER_BOUND ( 'NONE', #30175, .T. ) ;
#27755=B_SPLINE_CURVE_WITH_KNOTS ( 'NONE', 3,
 ( #1828, #6971, #20846, #3867 ),
 .UNSPECIFIED., .F., .F.,
 ( 4, 4 ),
 ( 3.022186913382060468E-07, 0.007932103869840216592 ),
 .UNSPECIFIED. ) ;
#27756=CARTESIAN_POINT ( 'NONE',  ( 32.60829997825920401, -13.18983524832148113, 35.60092001944722995 ) ) ;
#27764=AXIS2_PLACEMENT_3D ( 'NONE', #1218, #5585, #20225 ) ;
#27768=ORIENTED_EDGE ( 'NONE', *, *, #8631, .T. ) ;
#27800=CARTESIAN_POINT ( 'NONE',  ( 23.07500649350761179, -11.56036165373734725, 49.19141369487476112 ) ) ;
#27805=CARTESIAN_POINT ( 'NONE',  ( 33.01877980957529957, 12.12572312222181026, 39.84356070656652804 ) ) ;
#27820=B_SPLINE_CURVE_WITH_KNOTS ( 'NONE', 3,
 ( #18489, #20948, #22680, #6170 ),
 .UNSPECIFIED., .F., .F.,
 ( 4, 4 ),
 ( 2.143643656977390230E-07, 0.003421830178490235016 ),
 .UNSPECIFIED. ) ;
#27836=CARTESIAN_POINT ( 'NONE',  ( 38.04520357587708190, -9.701815779983750332, 31.93699797870259260 ) ) ;
#27871=CARTESIAN_POINT ( 'NONE',  ( 24.44496207165490631, -7.595930209050163029, 49.40206402021031096 ) ) ;
#27873=EDGE_CURVE ( 'NONE', #4107, #18044, #23718, .T. ) ;
#27891=VERTEX_POINT ( 'NONE', #9853 ) ;
#27899=CARTESIAN_POINT ( 'NONE',  ( 24.44496207165490631, -7.595930209050163029, 49.40206402021031096 ) ) ;
#27906=CARTESIAN_POINT ( 'NONE',  ( 4.677126025380961671, -39.24912351428227453, 34.80090346875809360 ) ) ;
#27910=EDGE_CURVE ( 'NONE', #19006, #10874, #7366, .T. ) ;
#27947=CARTESIAN_POINT ( 'NONE',  ( -8.552541667382493884, 38.37438965712765082, 27.50000000000000355 ) ) ;
#27980=CARTESIAN_POINT ( 'NONE',  ( 14.45970719238747115, -39.47880481153868004, 34.54750567515515769 ) ) ;
#27988=CARTESIAN_POINT ( 'NONE',  ( -8.318988986562537491, -36.57037096148668098, 37.50000000002251710 ) ) ;
#27993=CARTESIAN_POINT ( 'NONE',  ( -29.61203839202723032, 15.40012917324033381, 37.38016955275591613 ) ) ;
#28000=DIRECTION ( 'NONE',  ( 1.000000000000000000, 0.000000000000000000, 0.000000000000000000 ) ) ;
#28028=CARTESIAN_POINT ( 'NONE',  ( -27.03074382657074537, 6.449748410230984774, 42.96778633356043287 ) ) ;
#28042=CARTESIAN_POINT ( 'NONE',  ( 2.338573377552013888, -39.50000000000001421, 27.50000000000001066 ) ) ;
#28069=ADVANCED_FACE ( 'NONE', ( #11087 ), #23068, .F. ) ;
#28075=CARTESIAN_POINT ( 'NONE',  ( -34.83396020575241891, -10.30249279383514960, 34.80090346875805096 ) ) ;
#28086=CARTESIAN_POINT ( 'NONE',  ( 23.21352257770656990, 10.78826658734920230, 45.15942333309104129 ) ) ;
#28091=CARTESIAN_POINT ( 'NONE',  ( -29.06918585179853665, 23.33130127174517554, 27.50000000000000711 ) ) ;
#28095=DIRECTION ( 'NONE',  ( -0.000000000000000000, -0.000000000000000000, -1.000000000000000000 ) ) ;
#28099=B_SPLINE_CURVE_WITH_KNOTS ( 'NONE', 3,
 ( #8721, #18235, #27756, #29628 ),
 .UNSPECIFIED., .F., .F.,
 ( 4, 4 ),
 ( 2.143643656948718959E-07, 0.003421830178490221138 ),
 .UNSPECIFIED. ) ;
#28101=CARTESIAN_POINT ( 'NONE',  ( -35.13802340818978820, 8.772855875111229551, 34.58409965093399308 ) ) ;
#28103=CARTESIAN_POINT ( 'NONE',  ( 32.28307784207223108, 8.475829241206289666, 41.62281023987511475 ) ) ;
#28104=VERTEX_POINT ( 'NONE', #11232 ) ;
#28107=CARTESIAN_POINT ( 'NONE',  ( -4.281329142241829366, -42.25336671256035004, 28.86098669521330251 ) ) ;
#28109=VERTEX_POINT ( 'NONE', #20728 ) ;
#28122=VERTEX_POINT ( 'NONE', #30108 ) ;
#28128=DIRECTION ( 'NONE',  ( 0.9329908884337522190, 0.3598999890241700306, 0.000000000000000000 ) ) ;
#28132=CARTESIAN_POINT ( 'NONE',  ( 24.45718231057517400, -33.13439223474804862, 29.72618443979869696 ) ) ;
#28135=CARTESIAN_POINT ( 'NONE',  ( -33.42925964089141644, -11.06161099612212695, 35.54550565580013455 ) ) ;
#28154=CARTESIAN_POINT ( 'NONE',  ( -24.18487066411276487, 13.30660647122584983, 43.15349873716021278 ) ) ;
#28157=ORIENTED_EDGE ( 'NONE', *, *, #18141, .T. ) ;
#28170=CARTESIAN_POINT ( 'NONE',  ( -35.86518915568154142, 11.02596425420269100, 37.50000000003379341 ) ) ;
#28172=PLANE ( 'NONE',  #20818 ) ;
#28184=CARTESIAN_POINT ( 'NONE',  ( 25.41307773079512344, -6.523700759042262654, 48.76310947883586522 ) ) ;
#28187=LINE ( 'NONE', #30386, #23834 ) ;
#28194=EDGE_CURVE ( 'NONE', #18819, #2982, #2187, .T. ) ;
#28239=CARTESIAN_POINT ( 'NONE',  ( -31.54493124927535419, 19.07059040393068727, 27.50000000000000711 ) ) ;
#28259=CARTESIAN_POINT ( 'NONE',  ( 33.02695388770936802, 15.72686850277320936, 27.50000000000000355 ) ) ;
#28262=CARTESIAN_POINT ( 'NONE',  ( 0.000000000000000000, 42.50000000000000000, 27.50000000000000355 ) ) ;
#28290=CARTESIAN_POINT ( 'NONE',  ( 24.35970437652574816, -13.37404834226503958, -16.55003854064094426 ) ) ;
#28291=CARTESIAN_POINT ( 'NONE',  ( 12.47055468150928625, -35.37063655238940640, 37.50000000000014211 ) ) ;
#28296=VECTOR ( 'NONE', #4766, 1000.000000000000000 ) ;
#28319=CARTESIAN_POINT ( 'NONE',  ( -5.127072262013854242, -42.13114360820154047, 28.87158698979397897 ) ) ;
#28342=CARTESIAN_POINT ( 'NONE',  ( -35.58199486000248157, 17.45398116881282391, 34.79408014406299543 ) ) ;
#28343=ORIENTED_EDGE ( 'NONE', *, *, #25932, .T. ) ;
#28357=CARTESIAN_POINT ( 'NONE',  ( 26.58597676761596418, -6.321098805557485711, 47.67294373134342322 ) ) ;
#28362=CARTESIAN_POINT ( 'NONE',  ( -24.44496207165490276, 7.595930209050158588, -16.55003854064094426 ) ) ;
#28363=AXIS2_PLACEMENT_3D ( 'NONE', #16229, #28095, #25608 ) ;
#28365=ORIENTED_EDGE ( 'NONE', *, *, #17933, .F. ) ;
#28388=ORIENTED_EDGE ( 'NONE', *, *, #23926, .T. ) ;
#28390=CARTESIAN_POINT ( 'NONE',  ( 13.81384208584302975, -36.54172128922432705, 34.50000000000000000 ) ) ;
#28401=CARTESIAN_POINT ( 'NONE',  ( -26.44471942863318148, -26.80494974449361933, 27.50000000000000000 ) ) ;
#28409=EDGE_LOOP ( 'NONE', ( #23588, #23739, #17059, #17787 ) ) ;
#28414=CARTESIAN_POINT ( 'NONE',  ( 18.68937984944595954, -33.86068137868598171, 27.50000000000000000 ) ) ;
#28428=ORIENTED_EDGE ( 'NONE', *, *, #16501, .F. ) ;
#28434=CARTESIAN_POINT ( 'NONE',  ( -33.42925964089140933, 11.06161099612212695, 35.54550565580014876 ) ) ;
#28438=CARTESIAN_POINT ( 'NONE',  ( 38.33765298566224544, 8.216851622513988929, 32.02327563374863928 ) ) ;
#28445=( BOUNDED_SURFACE ( )  B_SPLINE_SURFACE ( 3, 2, ( 
 ( #27725, #8699, #18057 ),
 ( #6356, #1980, #13840 ),
 ( #11501, #23021, #25386 ),
 ( #29753, #13541, #4014 ),
 ( #11187, #1371, #8399 ),
 ( #27426, #6507, #20684 ),
 ( #4308, #30211, #25221 ),
 ( #6044, #15553, #3715 ),
 ( #11350, #20844, #13229 ),
 ( #10886, #27574, #6200 ),
 ( #15703, #3865, #9299 ),
 ( #6969, #9465, #14123 ),
 ( #14597, #23948, #23483 ),
 ( #9615, #28493, #18825 ),
 ( #18980, #2271, #21132 ),
 ( #11792, #24103, #5087 ),
 ( #2751, #14272, #7120 ),
 ( #20985, #4764, #16632 ),
 ( #26136, #16939, #13986 ),
 ( #23792, #30504, #19274 ),
 ( #16327, #28793, #25995 ),
 ( #4931, #2443, #16478 ),
 ( #2122, #9151, #11964 ),
 ( #11641, #18665, #7432 ),
 ( #16778, #28342, #21298 ),
 ( #4622, #26456, #14447 ),
 ( #23627, #21454, #30818 ),
 ( #2595, #25846, #28170 ),
 ( #7266, #98, #19125 ),
 ( #28641, #26295, #12113 ),
 ( #30651, #21612, #247 ),
 ( #6803, #9759, #4478 ),
 ( #19582, #24714, #22390 ),
 ( #10220, #12890, #8051 ),
 ( #2909, #26771, #14741 ),
 ( #15358, #19432, #24886 ),
 ( #5545, #5856, #26928 ),
 ( #15192, #7901, #8196 ),
 ( #17087, #15047, #12260 ),
 ( #29564, #7586, #10534 ),
 ( #17243, #5243, #24562 ),
 ( #17701, #29100, #28950 ),
 ( #26615, #5399, #404 ),
 ( #862, #19730, #20042 ),
 ( #3206, #12728, #24259 ),
 ( #22225, #10386, #12425 ),
 ( #27071, #3357, #21920 ),
 ( #548, #29416, #22068 ),
 ( #29257, #24412, #19901 ),
 ( #21765, #10071, #17554 ),
 ( #1026, #7741, #5697 ),
 ( #27219, #14905, #9919 ),
 ( #3054, #17408, #12577 ),
 ( #704, #25031, #18025 ),
 ( #6472, #29884, #8807 ),
 ( #6621, #16134, #3525 ),
 ( #3822, #8524, #8969 ),
 ( #27538, #15983, #1179 ),
 ( #4127, #25504, #13506 ),
 ( #20187, #6162, #25343 ),
 ( #13346, #1326, #22988 ),
 ( #23139, #20801, #20359 ),
 ( #15665, #25177, #27988 ),
 ( #6008, #13656, #27389 ),
 ( #10848, #1786, #22675 ),
 ( #18484, #20652, #22528 ) ),
 .UNSPECIFIED., .F., .F., .T. ) 
 B_SPLINE_SURFACE_WITH_KNOTS ( ( 4, 2, 2, 2, 2, 2, 2, 2, 2, 2, 2, 2, 2, 2, 2, 2, 2, 2, 2, 2, 2, 2, 2, 2, 2, 2, 2, 2, 2, 2, 2, 2, 4 ),
 ( 3, 3 ),
 ( 0.000000000000000000, 0.006029285522234034342, 0.009043928283351050645, 0.01205857104446806868, 0.01507321380558508499, 0.01658053518614359401, 0.01808785656670210129, 0.02411714208893613737, 0.02562446346949464465, 0.02713178485005315194, 0.03014642761117016997, 0.03617571313340420258, 0.03919035589452121715, 0.04220499865563823866, 0.04521964141675526017, 0.04672696279731376745, 0.04823428417787227473, 0.05426356970010630387, 0.05727821246122331844, 0.05878553384178182573, 0.06029285522234033995, 0.06632214074457437603, 0.06933678350569139059, 0.07084410488624989788, 0.07235142626680840516, 0.07838071178904243430, 0.08139535455015944887, 0.08290267593071795615, 0.08440999731127647732, 0.09043928283351052033, 0.09194660421406902762, 0.09345392559462753490, 0.09646856835574454947 ),
 ( 0.000000000000000000, 1.000000000000000000 ),
 .UNSPECIFIED. ) 
 GEOMETRIC_REPRESENTATION_ITEM ( )  RATIONAL_B_SPLINE_SURFACE ( (
 ( 1.000000000000000000, 0.8675023601337629175, 1.000000000000000000),
 ( 1.000000000000000000, 0.8658666847259426369, 1.000000000000000000),
 ( 1.000000000000000000, 0.8655958742315080778, 1.000000000000000000),
 ( 1.000000000000000000, 0.8671900595434904879, 1.000000000000000000),
 ( 1.000000000000000000, 0.8680562056017228079, 1.000000000000000000),
 ( 1.000000000000000000, 0.8704419788917913126, 1.000000000000000000),
 ( 1.000000000000000000, 0.8719392239578002135, 1.000000000000000000),
 ( 1.000000000000000000, 0.8754638309335783797, 1.000000000000000000),
 ( 1.000000000000000000, 0.8774913221368225713, 1.000000000000000000),
 ( 1.000000000000000000, 0.8808764947177999405, 1.000000000000000000),
 ( 1.000000000000000000, 0.8820622495001770869, 1.000000000000000000),
 ( 1.000000000000000000, 0.8845398562658981501, 1.000000000000000000),
 ( 1.000000000000000000, 0.8858356588747311466, 1.000000000000000000),
 ( 1.000000000000000000, 0.8924978076758027790, 1.000000000000000000),
 ( 1.000000000000000000, 0.8984086608255127393, 1.000000000000000000),
 ( 1.000000000000000000, 0.9060753982733059653, 1.000000000000000000),
 ( 1.000000000000000000, 0.9076229079092951180, 1.000000000000000000),
 ( 1.000000000000000000, 0.9107356538043366312, 1.000000000000000000),
 ( 1.000000000000000000, 0.9123045924019421715, 1.000000000000000000),
 ( 1.000000000000000000, 0.9169824489404084789, 1.000000000000000000),
 ( 1.000000000000000000, 0.9200684232435814014, 1.000000000000000000),
 ( 1.000000000000000000, 0.9291119025149430222, 1.000000000000000000),
 ( 1.000000000000000000, 0.9348565328406341912, 1.000000000000000000),
 ( 1.000000000000000000, 0.9425865537118557347, 1.000000000000000000),
 ( 1.000000000000000000, 0.9449872438562321175, 1.000000000000000000),
 ( 1.000000000000000000, 0.9493613651927652608, 1.000000000000000000),
 ( 1.000000000000000000, 0.9513387435488267485, 1.000000000000000000),
 ( 1.000000000000000000, 0.9548238729109979062, 1.000000000000000000),
 ( 1.000000000000000000, 0.9563316464886052470, 1.000000000000000000),
 ( 1.000000000000000000, 0.9582033662281566055, 1.000000000000000000),
 ( 1.000000000000000000, 0.9587622799799166984, 1.000000000000000000),
 ( 1.000000000000000000, 0.9597437750956563374, 1.000000000000000000),
 ( 1.000000000000000000, 0.9601664819861042144, 1.000000000000000000),
 ( 1.000000000000000000, 0.9619094554756278947, 1.000000000000000000),
 ( 1.000000000000000000, 0.9621362728652917973, 1.000000000000000000),
 ( 1.000000000000000000, 0.9607577752117092418, 1.000000000000000000),
 ( 1.000000000000000000, 0.9600123908336705147, 1.000000000000000000),
 ( 1.000000000000000000, 0.9584744574991911348, 1.000000000000000000),
 ( 1.000000000000000000, 0.9578918694617124530, 1.000000000000000000),
 ( 1.000000000000000000, 0.9565886671613721415, 1.000000000000000000),
 ( 1.000000000000000000, 0.9558692645217879980, 1.000000000000000000),
 ( 1.000000000000000000, 0.9519759472186718474, 1.000000000000000000),
 ( 1.000000000000000000, 0.9478928039660258209, 1.000000000000000000),
 ( 1.000000000000000000, 0.9406739587686179238, 1.000000000000000000),
 ( 1.000000000000000000, 0.9380850758978200865, 1.000000000000000000),
 ( 1.000000000000000000, 0.9339721408369989764, 1.000000000000000000),
 ( 1.000000000000000000, 0.9325593384373154215, 1.000000000000000000),
 ( 1.000000000000000000, 0.9296829639154353675, 1.000000000000000000),
 ( 1.000000000000000000, 0.9282220600982826753, 1.000000000000000000),
 ( 1.000000000000000000, 0.9208300713421492256, 1.000000000000000000),
 ( 1.000000000000000000, 0.9146367548417139171, 1.000000000000000000),
 ( 1.000000000000000000, 0.9054116939033787226, 1.000000000000000000),
 ( 1.000000000000000000, 0.9023473709286883304, 1.000000000000000000),
 ( 1.000000000000000000, 0.8978322988697580165, 1.000000000000000000),
 ( 1.000000000000000000, 0.8963369152402574924, 1.000000000000000000),
 ( 1.000000000000000000, 0.8934211100373304903, 1.000000000000000000),
 ( 1.000000000000000000, 0.8919972686373036641, 1.000000000000000000),
 ( 1.000000000000000000, 0.8850723860929040621, 1.000000000000000000),
 ( 1.000000000000000000, 0.8801508607758546932, 1.000000000000000000),
 ( 1.000000000000000000, 0.8751780230577477226, 1.000000000000000000),
 ( 1.000000000000000000, 0.8742426755642516145, 1.000000000000000000),
 ( 1.000000000000000000, 0.8725019882397289095, 1.000000000000000000),
 ( 1.000000000000000000, 0.8716945872086134806, 1.000000000000000000),
 ( 1.000000000000000000, 0.8695096448583727877, 1.000000000000000000),
 ( 1.000000000000000000, 0.8683626000225895814, 1.000000000000000000),
 ( 1.000000000000000000, 0.8675417673879197711, 1.000000000000000000) ) ) 
 REPRESENTATION_ITEM ( '' )  SURFACE ( )  );
#28451=CARTESIAN_POINT ( 'NONE',  ( -31.22486525274646851, -15.32888848509419510, 35.97296397489743924 ) ) ;
#28473=CARTESIAN_POINT ( 'NONE',  ( 33.36623411648999848, -9.470136927103574465, 36.07330332824747643 ) ) ;
#28481=CARTESIAN_POINT ( 'NONE',  ( -34.70577939416727276, 10.49309206033987785, 34.49999999999999289 ) ) ;
#28493=CARTESIAN_POINT ( 'NONE',  ( -21.00291486166312183, 35.92820678882968366, 34.50839795287551937 ) ) ;
#28499=DIRECTION ( 'NONE',  ( -0.000000000000000000, -0.000000000000000000, 1.000000000000000000 ) ) ;
#28502=CARTESIAN_POINT ( 'NONE',  ( 24.57973596967192265, -7.302173446879558938, 49.35895363830199045 ) ) ;
#28514=DIRECTION ( 'NONE',  ( 0.000000000000000000, 0.000000000000000000, 1.000000000000000000 ) ) ;
#28520=ORIENTED_EDGE ( 'NONE', *, *, #28852, .T. ) ;
#28524=CARTESIAN_POINT ( 'NONE',  ( -25.41307773079511634, 6.523700759042264430, 48.76310947883596469 ) ) ;
#28532=CARTESIAN_POINT ( 'NONE',  ( -17.27847337688485396, -38.19802013284401454, 29.22704955593633613 ) ) ;
#28540=B_SPLINE_CURVE_WITH_KNOTS ( 'NONE', 3,
 ( #8817, #27544, #18343, #1795, #16142, #6172, #4277, #23308, #20950, #10855, #9117, #18639, #15524, #20365 ),
 .UNSPECIFIED., .F., .F.,
 ( 4, 2, 2, 2, 2, 2, 4 ),
 ( 2.108697328626194806E-07, 0.0004867403590529698022, 0.0009732698483730769980, 0.001459799337693184085, 0.001946328827013291390, 0.002919387805653492120, 0.003892446784293693285 ),
 .UNSPECIFIED. ) ;
#28546=B_SPLINE_CURVE_WITH_KNOTS ( 'NONE', 3,
 ( #7639, #17302, #15109, #27134 ),
 .UNSPECIFIED., .F., .F.,
 ( 4, 4 ),
 ( 2.143643656964904170E-07, 0.003421830178490233715 ),
 .UNSPECIFIED. ) ;
#28547=DIRECTION ( 'NONE',  ( 0.000000000000000000, 0.000000000000000000, 1.000000000000000000 ) ) ;
#28550=CARTESIAN_POINT ( 'NONE',  ( -33.04966240345561346, 15.66936333904344814, 27.50000000000001421 ) ) ;
#28553=CARTESIAN_POINT ( 'NONE',  ( -11.01465109972504486, -37.62049097135311371, 34.49999999999999289 ) ) ;
#28554=FACE_OUTER_BOUND ( 'NONE', #14083, .T. ) ;
#28565=CARTESIAN_POINT ( 'NONE',  ( 4.958664261655640892, 39.14709335570276494, 27.50000000000001066 ) ) ;
#28584=CARTESIAN_POINT ( 'NONE',  ( -33.48612972047447300, 10.91418318924902131, 35.53782825235610687 ) ) ;
#28585=ORIENTED_EDGE ( 'NONE', *, *, #11116, .T. ) ;
#28588=CARTESIAN_POINT ( 'NONE',  ( 35.80460862680673273, 16.89914958172166237, 31.37043939660702563 ) ) ;
#28600=PRODUCT_DEFINITION_SHAPE ( 'NONE', 'NONE',  #3621 ) ;
#28604=ADVANCED_FACE ( 'NONE', ( #11863 ), #21362, .F. ) ;
#28617=DIRECTION ( 'NONE',  ( -0.000000000000000000, -0.000000000000000000, -1.000000000000000000 ) ) ;
#28636=EDGE_CURVE ( 'NONE', #20389, #17339, #10875, .T. ) ;
#28641=CARTESIAN_POINT ( 'NONE',  ( -38.33685850190697408, 7.830772188364141684, 32.02836762638165169 ) ) ;
#28645=CARTESIAN_POINT ( 'NONE',  ( 33.48319591361583036, 9.771272583783430221, 35.87764403311519601 ) ) ;
#28708=CARTESIAN_POINT ( 'NONE',  ( -34.70577939417217550, -10.49309206032214270, 34.49999999999999289 ) ) ;
#28711=EDGE_LOOP ( 'NONE', ( #24376, #3521, #7548, #6861 ) ) ;
#28721=CARTESIAN_POINT ( 'NONE',  ( 33.25228913575067224, 15.14457679224870823, 27.50000000000000711 ) ) ;
#28744=CARTESIAN_POINT ( 'NONE',  ( 28.40824562282756816, 24.48677906707029095, 37.49999999999575095 ) ) ;
#28750=CARTESIAN_POINT ( 'NONE',  ( -23.72453467988983178, -12.99099554674205947, 43.70890687484121173 ) ) ;
#28771=CARTESIAN_POINT ( 'NONE',  ( -4.776122516674677878E-15, -42.50000000000000000, 27.50000000000000355 ) ) ;
#28775=CARTESIAN_POINT ( 'NONE',  ( -32.19782014694307293, -14.25394737442115733, 35.54550565580014876 ) ) ;
#28793=CARTESIAN_POINT ( 'NONE',  ( -29.63644584941609139, 27.66395999911765458, 34.56506848433971868 ) ) ;
#28805=EDGE_CURVE ( 'NONE', #18778, #28122, #24419, .T. ) ;
#28841=EDGE_LOOP ( 'NONE', ( #11588, #2910, #5882, #8453, #961, #20933 ) ) ;
#28843=CARTESIAN_POINT ( 'NONE',  ( 28.97452988725117962, 28.45570922648237300, 30.21020218777692889 ) ) ;
#28852=EDGE_CURVE ( 'NONE', #12760, #10675, #17771, .T. ) ;
#28857=EDGE_LOOP ( 'NONE', ( #30680, #28428, #11881, #27147, #30110, #665, #21946, #8797, #20546 ) ) ;
#28878=CYLINDRICAL_SURFACE ( 'NONE', #11378, 1.999999999999998224 ) ;
#28888=CARTESIAN_POINT ( 'NONE',  ( 29.61203839202722676, 15.40012917324034092, 41.62281023987512185 ) ) ;
#28901=CARTESIAN_POINT ( 'NONE',  ( 33.58313301488747271, 16.73358698008457424, 37.50000000006255618 ) ) ;
#28917=CARTESIAN_POINT ( 'NONE',  ( -25.23650299772496197, 28.24517122938463842, 34.50000000000000000 ) ) ;
#28950=CARTESIAN_POINT ( 'NONE',  ( -35.18685215751978745, -13.22180849084768006, 37.49999999986729193 ) ) ;
#28992=DIRECTION ( 'NONE',  ( -0.3598999890241648680, -0.9329908884337543284, 0.000000000000000000 ) ) ;
#28999=ORIENTED_EDGE ( 'NONE', *, *, #26738, .T. ) ;
#29011=CARTESIAN_POINT ( 'NONE',  ( -17.83717022821180009, -34.31216324508217497, 34.50000000000000000 ) ) ;
#29013=DIRECTION ( 'NONE',  ( 1.000000000000000000, 0.000000000000000000, 0.000000000000000000 ) ) ;
#29033=CARTESIAN_POINT ( 'NONE',  ( 31.46019086465472014, 15.19107625323260891, 40.06435153370524915 ) ) ;
#29047=CARTESIAN_POINT ( 'NONE',  ( -4.375757216953428294E-15, -39.50000000000000000, 37.50000000000000000 ) ) ;
#29049=CARTESIAN_POINT ( 'NONE',  ( 38.97222564111406484, -2.062036942600702805, 32.22331656435463287 ) ) ;
#29064=CARTESIAN_POINT ( 'NONE',  ( -2.025933774932175968, 39.50000000000001421, 34.50000000000000000 ) ) ;
#29095=VECTOR ( 'NONE', #6955, 1000.000000000000000 ) ;
#29100=CARTESIAN_POINT ( 'NONE',  ( -37.05526867389234980, -13.52123220197743336, 34.89587700162063300 ) ) ;
#29111=EDGE_CURVE ( 'NONE', #13000, #13876, #9596, .T. ) ;
#29118=CARTESIAN_POINT ( 'NONE',  ( 0.000000000000000000, 42.50000000000000000, 32.33822642395377045 ) ) ;
#29120=DIRECTION ( 'NONE',  ( -0.000000000000000000, -0.000000000000000000, 1.000000000000000000 ) ) ;
#29146=CARTESIAN_POINT ( 'NONE',  ( -21.56949286799591903, -35.43467754613438814, 29.49548763488747483 ) ) ;
#29167=ORIENTED_EDGE ( 'NONE', *, *, #20624, .F. ) ;
#29172=CARTESIAN_POINT ( 'NONE',  ( -24.57973596967191554, 7.302173446879558050, 45.11631295118280605 ) ) ;
#29197=EDGE_CURVE ( 'NONE', #1784, #30101, #21062, .T. ) ;
#29200=CARTESIAN_POINT ( 'NONE',  ( 4.963855673496207821, 42.15448181593355059, 34.60401223484481648 ) ) ;
#29206=ORIENTED_EDGE ( 'NONE', *, *, #21956, .F. ) ;
#29208=DIRECTION ( 'NONE',  ( -0.000000000000000000, -0.000000000000000000, 1.000000000000000000 ) ) ;
#29236=CARTESIAN_POINT ( 'NONE',  ( 33.56327786402393798, -10.22184951998668012, 35.67222448829685533 ) ) ;
#29257=CARTESIAN_POINT ( 'NONE',  ( -31.96377083499153571, -24.36009066984772531, 30.63716218392069024 ) ) ;
#29288=CARTESIAN_POINT ( 'NONE',  ( -27.60655220535237575, -25.35568602214586065, 27.50000000000000355 ) ) ;
#29290=B_SPLINE_CURVE_WITH_KNOTS ( 'NONE', 3,
 ( #3135, #1103, #22151, #8128 ),
 .UNSPECIFIED., .F., .F.,
 ( 4, 4 ),
 ( 2.143643656964903641E-07, 0.003421830178490235450 ),
 .UNSPECIFIED. ) ;
#29295=VERTEX_POINT ( 'NONE', #29534 ) ;
#29304=CARTESIAN_POINT ( 'NONE',  ( 26.40719054689828837, 31.30341782987545329, 29.91384141721222889 ) ) ;
#29310=CARTESIAN_POINT ( 'NONE',  ( -23.69684009293500893, 33.86367947567046599, 29.65129610998314647 ) ) ;
#29313=VERTEX_POINT ( 'NONE', #14872 ) ;
#29315=CARTESIAN_POINT ( 'NONE',  ( 27.19231046524321371, -25.90237096470084310, 34.50000000000000711 ) ) ;
#29339=CONICAL_SURFACE ( 'NONE', #7430, 35.37867965644036872, 0.7853981633974500554 ) ;
#29346=CARTESIAN_POINT ( 'NONE',  ( 31.10910608030087943, 19.98124338977578773, 34.49999999999999289 ) ) ;
#29347=CARTESIAN_POINT ( 'NONE',  ( -11.52197458429825083, 37.50933785548062360, 34.80090346875805096 ) ) ;
#29350=CARTESIAN_POINT ( 'NONE',  ( -11.39115782160862977, -40.65273190043797058, 29.00210455454194047 ) ) ;
#29352=CARTESIAN_POINT ( 'NONE',  ( -24.75988009833579184, -7.043597625963917253, 49.25816067347040672 ) ) ;
#29357=DIRECTION ( 'NONE',  ( 1.000000000000000000, 0.000000000000000000, 0.000000000000000000 ) ) ;
#29366=CARTESIAN_POINT ( 'NONE',  ( 16.56282882398535250, 33.64935822775603924, 37.49999999998171063 ) ) ;
#29370=CARTESIAN_POINT ( 'NONE',  ( -24.02316098943739675, -13.21662147465773707, 43.33855891335688426 ) ) ;
#29378=CARTESIAN_POINT ( 'NONE',  ( -34.70577939416727276, 10.49309206033987785, 34.49999999999999289 ) ) ;
#29416=CARTESIAN_POINT ( 'NONE',  ( -32.07676738547140616, -24.18760485068483135, 34.63128111633764661 ) ) ;
#29436=DIRECTION ( 'NONE',  ( -0.000000000000000000, -0.000000000000000000, -1.000000000000000000 ) ) ;
#29444=CARTESIAN_POINT ( 'NONE',  ( -35.99780421875948377, -2.509863319654308089, 27.50000000000000000 ) ) ;
#29457=DIRECTION ( 'NONE',  ( -0.000000000000000000, -0.000000000000000000, 1.000000000000000000 ) ) ;
#29459=B_SPLINE_CURVE_WITH_KNOTS ( 'NONE', 3,
 ( #1169, #20645, #1321, #10676 ),
 .UNSPECIFIED., .F., .F.,
 ( 4, 4 ),
 ( 3.018024802580205417E-07, 0.007932103453629116285 ),
 .UNSPECIFIED. ) ;
#29461=CARTESIAN_POINT ( 'NONE',  ( 29.78057599403043909, 27.44970389380054243, 30.31536403417277015 ) ) ;
#29465=CARTESIAN_POINT ( 'NONE',  ( -35.59958042135278333, -17.54967582489527445, 31.31518679243729864 ) ) ;
#29467=CARTESIAN_POINT ( 'NONE',  ( -29.61203839202723032, -15.40012917324033381, 41.62281023987518580 ) ) ;
#29500=CARTESIAN_POINT ( 'NONE',  ( 0.000000000000000000, 39.50000000000000000, 34.80090346875804386 ) ) ;
#29502=CARTESIAN_POINT ( 'NONE',  ( 32.06725342158286907, 14.54034564589948531, 39.79052675593687383 ) ) ;
#29505=CARTESIAN_POINT ( 'NONE',  ( 24.75988009833579540, 7.043597625963922582, 49.25816067347034277 ) ) ;
#29507=CARTESIAN_POINT ( 'NONE',  ( 33.55235357430897380, 10.58403138555777900, 35.57544210944276841 ) ) ;
#29516=B_SPLINE_CURVE_WITH_KNOTS ( 'NONE', 3,
 ( #15181, #12877, #5845, #22376, #6146, #24875, #10671, #20177, #20030, #13172, #22665, #22512, #15652, #25165 ),
 .UNSPECIFIED., .F., .F.,
 ( 4, 2, 2, 2, 2, 2, 4 ),
 ( 2.111077618484504239E-07, 0.0004668847438969953110, 0.0009335583800321421710, 0.001400232016167289248, 0.001866905652302435891, 0.002800252924572717468, 0.003733600196842999479 ),
 .UNSPECIFIED. ) ;
#29520=CARTESIAN_POINT ( 'NONE',  ( 25.18096005886327760, 6.640581704039639988, 44.71664046397091852 ) ) ;
#29521=CARTESIAN_POINT ( 'NONE',  ( -19.50000000000000711, 1.387778780781445676E-14, 62.49999999999999289 ) ) ;
#29531=CARTESIAN_POINT ( 'NONE',  ( -27.82441128074781744, 25.08107326869593479, 34.50000000000000000 ) ) ;
#29534=CARTESIAN_POINT ( 'NONE',  ( -33.42925964089141644, -11.06161099612212695, 39.78814634291941843 ) ) ;
#29564=CARTESIAN_POINT ( 'NONE',  ( -38.03082308345415896, -9.438271779104216108, 31.93948111368219500 ) ) ;
#29565=VERTEX_POINT ( 'NONE', #5484 ) ;
#29574=CARTESIAN_POINT ( 'NONE',  ( 29.61203839202723032, 15.40012917324034092, 37.38016955275583797 ) ) ;
#29590=EDGE_CURVE ( 'NONE', #8115, #20027, #30366, .T. ) ;
#29596=ADVANCED_FACE ( 'NONE', ( #17170 ), #711, .T. ) ;
#29628=CARTESIAN_POINT ( 'NONE',  ( 32.19782014694308003, -14.25394737442115201, 35.54550565580006349 ) ) ;
#29631=( BOUNDED_SURFACE ( )  B_SPLINE_SURFACE ( 3, 1, ( 
 ( #29118, #26944 ),
 ( #15063, #24577 ),
 ( #5103, #16952 ),
 ( #5415, #24277 ) ),
 .UNSPECIFIED., .F., .F., .T. ) 
 B_SPLINE_SURFACE_WITH_KNOTS ( ( 4, 4 ),
 ( 2, 2 ),
 ( 0.000000000000000000, 1.000000000000000000 ),
 ( 0.000000000000000000, 1.000000000000000000 ),
 .UNSPECIFIED. ) 
 GEOMETRIC_REPRESENTATION_ITEM ( )  RATIONAL_B_SPLINE_SURFACE ( (
 ( 1.000000000000000000, 1.000000000000000000),
 ( 0.3333333333333333703, 0.3333333333333333703),
 ( 0.3333333333333333703, 0.3333333333333333703),
 ( 1.000000000000000000, 1.000000000000000000) ) ) 
 REPRESENTATION_ITEM ( '' )  SURFACE ( )  );
#29649=CARTESIAN_POINT ( 'NONE',  ( 32.60641126234700238, 8.625635766581057240, 41.27204228840735567 ) ) ;
#29659=DIRECTION ( 'NONE',  ( -0.7071067811865487940, -8.659560562354948882E-17, -0.7071067811865463515 ) ) ;
#29663=CARTESIAN_POINT ( 'NONE',  ( -23.59115238065502851, -12.85789229732232464, 48.13252386464831289 ) ) ;
#29668=CARTESIAN_POINT ( 'NONE',  ( 7.711002885858497358, 41.77047323054696193, 34.59400228303246649 ) ) ;
#29674=AXIS2_PLACEMENT_3D ( 'NONE', #4562, #5180, #11906 ) ;
#29693=VECTOR ( 'NONE', #29436, 1000.000000000000000 ) ;
#29703=CARTESIAN_POINT ( 'NONE',  ( -4.272706734781662519, -37.25579118953926638, 37.50000000000000000 ) ) ;
#29707=VECTOR ( 'NONE', #1992, 1000.000000000000000 ) ;
#29711=B_SPLINE_CURVE_WITH_KNOTS ( 'NONE', 3,
 ( #11689, #26035, #23675, #2321, #11848, #29350, #2486, #19022, #28532, #2634, #29146, #27124, #12477, #9975, #10113, #24144, #22273, #21968, #14952, #24463, #8249, #19623, #12938, #29465, #7781, #17291, #7951, #26825, #918, #15097, #10264, #17132, #26655, #10585, #24615, #22431, #5449, #457, #3107, #12626, #12311, #7626, #19778, #22117, #24768, #2961, #3247, #5748, #744, #24310, #29310, #12773, #598, #17455, #26978, #5604, #8100, #19479, #17757, #10434, #17606, #19948, #20099, #15239 ),
 .UNSPECIFIED., .F., .F.,
 ( 4, 2, 2, 2, 2, 2, 2, 2, 2, 2, 2, 2, 2, 2, 2, 2, 2, 2, 2, 2, 2, 2, 2, 2, 2, 2, 2, 2, 2, 2, 2, 4 ),
 ( 0.1344761468983755315, 0.1383589492301900981, 0.1403003503960973675, 0.1422417515620046369, 0.1500073562256337700, 0.1538901585574483366, 0.1558315597233556060, 0.1577729608892629032, 0.1655385655528919808, 0.1694213678847065196, 0.1713627690506138168, 0.1733041702165210862, 0.1810697748801501916, 0.1849525772119647304, 0.1888353795437792970, 0.1966009842074084024, 0.1985423853733156718, 0.2004837865392229690, 0.2043665888710375356, 0.2121321935346666410, 0.2160149958664812075, 0.2198977981982957464, 0.2237806005301102852, 0.2257220016960175824, 0.2276634028619248240, 0.2354290075255539016, 0.2393118098573684405, 0.2431946121891829793, 0.2509602168528121124, 0.2529016180187193541, 0.2548430191846266513, 0.2587258215164411901 ),
 .UNSPECIFIED. ) ;
#29727=CARTESIAN_POINT ( 'NONE',  ( -22.50000000000000711, 1.387778780781445676E-14, 62.49999999999999289 ) ) ;
#29734=ORIENTED_EDGE ( 'NONE', *, *, #20259, .T. ) ;
#29753=CARTESIAN_POINT ( 'NONE',  ( -4.704423459274687858, 42.21704346353420334, 28.86412666609725264 ) ) ;
#29768=B_SPLINE_CURVE_WITH_KNOTS ( 'NONE', 3,
 ( #451, #12473, #2955, #19473, #22268, #26650, #26493, #23983, #16830, #29304, #21963, #22113, #28843, #29461, #26345, #2630, #14947, #591, #10109, #12152, #7776, #7946, #21651, #9808, #26973, #12767, #24458, #3101, #7477, #17286, #12619, #10259, #17919, #5901, #27583, #27737, #27270, #22427, #23031, #5742, #1680, #20241, #11197, #11047, #10581, #20548, #1071, #25232, #15402, #30069, #24927, #6210, #13551, #3878, #27119, #1384, #17750, #15713, #3563, #8708, #12934, #6053 ),
 .UNSPECIFIED., .F., .F.,
 ( 4, 2, 2, 2, 2, 2, 2, 2, 2, 2, 2, 2, 2, 2, 2, 2, 2, 2, 2, 2, 2, 2, 2, 2, 2, 2, 2, 2, 2, 2, 4 ),
 ( 0.005072925043687738153, 0.01283750835505231488, 0.01671980001073460065, 0.02060209166641688988, 0.02836667497778148916, 0.03224896663346377840, 0.03419011246130493342, 0.03613125828914608151, 0.04389584160051068773, 0.04777813325619299084, 0.05166042491187529395, 0.05942500822323989323, 0.06330729987892219635, 0.06524844570676334443, 0.06718959153460449252, 0.07495417484596912649, 0.07883646650165142267, 0.08077761232949258463, 0.08271875815733373272, 0.09048334146869832506, 0.09242448729653947315, 0.09436563312438060735, 0.09824792478006287577, 0.1021302164357451442, 0.1040713622635862923, 0.1060125080914274404, 0.1137770914027920188, 0.1157182372306331808, 0.1176593830584743428, 0.1215416747141566389, 0.1293062580255212313 ),
 .UNSPECIFIED. ) ;
#29781=CARTESIAN_POINT ( 'NONE',  ( 31.18890335284658022, 19.89223002944920538, 34.80090346875810070 ) ) ;
#29798=DIRECTION ( 'NONE',  ( -0.9329908884337538844, 0.3598999890241658117, 0.000000000000000000 ) ) ;
#29814=CARTESIAN_POINT ( 'NONE',  ( 33.36692087966583387, 9.471517865689168758, 40.31490688621818208 ) ) ;
#29817=CARTESIAN_POINT ( 'NONE',  ( -28.55068628633583216, -24.19494186940697134, 34.80090346875804386 ) ) ;
#29843=CARTESIAN_POINT ( 'NONE',  ( -33.56615453960540663, 10.45399542313511354, 39.84392849731690234 ) ) ;
#29855=VECTOR ( 'NONE', #29659, 1000.000000000000000 ) ;
#29860=DIRECTION ( 'NONE',  ( 0.000000000000000000, 0.000000000000000000, 1.000000000000000000 ) ) ;
#29865=CARTESIAN_POINT ( 'NONE',  ( -24.03448224033878944, -8.660042335149837456, 49.47829057475703252 ) ) ;
#29884=CARTESIAN_POINT ( 'NONE',  ( -22.32897562208770026, -34.85472879511701194, 34.50814406507193155 ) ) ;
#29892=CARTESIAN_POINT ( 'NONE',  ( 31.79204601741444236, 14.90874471747208219, 35.64345580000760805 ) ) ;
#29900=CARTESIAN_POINT ( 'NONE',  ( 35.99999999999969447, -0.8865895960784948571, 34.75735931288063085 ) ) ;
#29915=CARTESIAN_POINT ( 'NONE',  ( -31.10273980501929003, -15.38400267427140022, 36.05808397467838233 ) ) ;
#29947=CARTESIAN_POINT ( 'NONE',  ( -27.03074382657074537, 6.449748410230984774, 47.21042702067971675 ) ) ;
#29955=ORIENTED_EDGE ( 'NONE', *, *, #27313, .F. ) ;
#29985=CARTESIAN_POINT ( 'NONE',  ( -32.68377466358848693, -8.668986135640256663, 36.94359686629218942 ) ) ;
#30012=ORIENTED_EDGE ( 'NONE', *, *, #6123, .T. ) ;
#30015=CARTESIAN_POINT ( 'NONE',  ( 34.55425493108410251, -14.62473873825366688, 37.50000000006821210 ) ) ;
#30023=ORIENTED_EDGE ( 'NONE', *, *, #27873, .T. ) ;
#30027=CARTESIAN_POINT ( 'NONE',  ( -32.19782014694307293, -14.25394737442115733, 39.78814634291943264 ) ) ;
#30030=CARTESIAN_POINT ( 'NONE',  ( 31.22647667302025454, -15.32805873036034860, 40.21452297286836597 ) ) ;
#30035=CARTESIAN_POINT ( 'NONE',  ( -32.19782014694307293, -14.25394737442115733, 39.78814634291943264 ) ) ;
#30063=CARTESIAN_POINT ( 'NONE',  ( 28.78283879316666471, -7.125616703334846314, 45.34931131770218826 ) ) ;
#30069=CARTESIAN_POINT ( 'NONE',  ( 22.62972083932141487, -34.62032468731402446, 29.57672015196555293 ) ) ;
#30081=CARTESIAN_POINT ( 'NONE',  ( 15.85884089648733131, 35.55173462727347555, 27.50000000000001066 ) ) ;
#30092=B_SPLINE_CURVE_WITH_KNOTS ( 'NONE', 3,
 ( #15960, #4100, #13482, #22963 ),
 .UNSPECIFIED., .F., .F.,
 ( 4, 4 ),
 ( 2.143643656948718959E-07, 0.003421830178490221138 ),
 .UNSPECIFIED. ) ;
#30099=LINE ( 'NONE', #13874, #21874 ) ;
#30100=PRODUCT_DEFINITION_CONTEXT ( 'detailed design', #5613, 'design' ) ;
#30101=VERTEX_POINT ( 'NONE', #403 ) ;
#30107=CARTESIAN_POINT ( 'NONE',  ( -4.677126025380971441, -39.24912351428226742, 34.80090346875804386 ) ) ;
#30108=CARTESIAN_POINT ( 'NONE',  ( 33.56327786402390245, -10.34181101807379477, 39.87954049117192312 ) ) ;
#30110=ORIENTED_EDGE ( 'NONE', *, *, #21160, .F. ) ;
#30123=CARTESIAN_POINT ( 'NONE',  ( 35.13669516613780530, 8.778141986578262390, 34.58384122122917148 ) ) ;
#30125=CARTESIAN_POINT ( 'NONE',  ( 23.44182307864140569, -12.68276878097691807, 48.34755156432018453 ) ) ;
#30135=CARTESIAN_POINT ( 'NONE',  ( -32.28307784207223108, -8.475829241206282560, 37.38016955275590902 ) ) ;
#30146=CARTESIAN_POINT ( 'NONE',  ( -32.06827542805550024, 14.53851282002520762, 39.79035104390202804 ) ) ;
#30161=CARTESIAN_POINT ( 'NONE',  ( 36.51087454057529413, -15.00302545122030295, 34.85625572976320541 ) ) ;
#30170=EDGE_CURVE ( 'NONE', #19220, #3711, #20041, .T. ) ;
#30175=EDGE_LOOP ( 'NONE', ( #24656, #1336, #17045, #718 ) ) ;
#30201=( NAMED_UNIT ( * ) PLANE_ANGLE_UNIT ( ) SI_UNIT ( $, .RADIAN. ) );
#30211=CARTESIAN_POINT ( 'NONE',  ( -10.00384078742051663, 41.10499445384696315, 34.57841144790000953 ) ) ;
#30212=ORIENTED_EDGE ( 'NONE', *, *, #19663, .T. ) ;
#30219=CARTESIAN_POINT ( 'NONE',  ( 24.44496207165490631, -7.595930209050163029, 45.15942333309103418 ) ) ;
#30229=AXIS2_PLACEMENT_3D ( 'NONE', #6812, #1681, #20695 ) ;
#30232=CARTESIAN_POINT ( 'NONE',  ( 23.69412710310942316, 29.84645176427128277, 27.50000000000000355 ) ) ;
#30236=B_SPLINE_CURVE_WITH_KNOTS ( 'NONE', 3,
 ( #30035, #9272, #20662, #13667 ),
 .UNSPECIFIED., .F., .F.,
 ( 4, 4 ),
 ( 2.143643656964903906E-07, 0.003421830178490235450 ),
 .UNSPECIFIED. ) ;
#30242=CARTESIAN_POINT ( 'NONE',  ( 23.44138668973443984, 12.68271180600415882, 48.34797144684549863 ) ) ;
#30248=DIRECTION ( 'NONE',  ( -0.000000000000000000, -0.000000000000000000, 1.000000000000000000 ) ) ;
#30250=ORIENTED_EDGE ( 'NONE', *, *, #10939, .F. ) ;
#30277=CARTESIAN_POINT ( 'NONE',  ( 24.35970437652574816, -13.37404834226503958, 42.96778633356033339 ) ) ;
#30306=DIRECTION ( 'NONE',  ( -0.000000000000000000, -0.000000000000000000, 1.000000000000000000 ) ) ;
#30314=CARTESIAN_POINT ( 'NONE',  ( 21.45876801738695860, -30.77697269628944809, 37.49999999998526334 ) ) ;
#30315=ADVANCED_FACE ( 'NONE', ( #5855 ), #13037, .F. ) ;
#30317=ORIENTED_EDGE ( 'NONE', *, *, #27178, .F. ) ;
#30325=EDGE_CURVE ( 'NONE', #3241, #19329, #6168, .T. ) ;
#30348=DIRECTION ( 'NONE',  ( 0.000000000000000000, 0.000000000000000000, 1.000000000000000000 ) ) ;
#30352=ORIENTED_EDGE ( 'NONE', *, *, #16543, .T. ) ;
#30366=B_SPLINE_CURVE_WITH_KNOTS ( 'NONE', 3,
 ( #26691, #12815, #3288, #5946, #22005, #639 ),
 .UNSPECIFIED., .F., .F.,
 ( 4, 2, 4 ),
 ( 0.01057608626846272791, 0.01589305904739927652, 0.02121003182633582687 ),
 .UNSPECIFIED. ) ;
#30386=CARTESIAN_POINT ( 'NONE',  ( 35.37867965644032608, 1.387778780781445676E-14, 35.37867965644034740 ) ) ;
#30391=CARTESIAN_POINT ( 'NONE',  ( 9.268856789657281325, -38.25380398711768493, 34.80090346875808649 ) ) ;
#30416=VERTEX_POINT ( 'NONE', #18273 ) ;
#30429=CARTESIAN_POINT ( 'NONE',  ( 27.86235613436988245, -14.72519157938688927, 39.24389099736748676 ) ) ;
#30430=CARTESIAN_POINT ( 'NONE',  ( 23.11727550875142612, -11.99039815441031465, 48.95928115119115631 ) ) ;
#30441=ORIENTED_EDGE ( 'NONE', *, *, #22907, .F. ) ;
#30448=VERTEX_POINT ( 'NONE', #23084 ) ;
#30450=B_SPLINE_CURVE_WITH_KNOTS ( 'NONE', 3,
 ( #26619, #16942, #14745, #4935, #28645, #14450, #5246, #26300, #9619, #14603, #23952, #24264, #4627, #25999 ),
 .UNSPECIFIED., .F., .F.,
 ( 4, 2, 2, 2, 2, 2, 4 ),
 ( 0.0007411796533686788348, 0.001115232222424166831, 0.001489284791479654826, 0.001863337360535142822, 0.002237389929590630818, 0.002985495067701606810, 0.003733600205812582801 ),
 .UNSPECIFIED. ) ;
#30452=ORIENTED_EDGE ( 'NONE', *, *, #10521, .T. ) ;
#30460=CARTESIAN_POINT ( 'NONE',  ( 24.13122067046371910, -33.41988417744658335, 34.50846293216257266 ) ) ;
#30472=CARTESIAN_POINT ( 'NONE',  ( 30.74201181684196982, -15.50830195949553492, 40.56825029441215236 ) ) ;
#30480=ORIENTED_EDGE ( 'NONE', *, *, #22660, .T. ) ;
#30504=CARTESIAN_POINT ( 'NONE',  ( -28.80398144066251831, 28.69005184980560230, 34.54961338325146869 ) ) ;
#30512=CARTESIAN_POINT ( 'NONE',  ( -26.81381729043377504, 6.366069288663346093, 43.19821070580857025 ) ) ;
#30521=DIRECTION ( 'NONE',  ( -0.000000000000000000, -0.000000000000000000, 1.000000000000000000 ) ) ;
#30533=B_SPLINE_CURVE_WITH_KNOTS ( 'NONE', 3,
 ( #9881, #29064, #24681, #24529, #24379, #2864, #22190, #3322, #519, #21887, #824, #21721, #12853, #22351, #17519, #26891, #19858, #8018, #28917, #17203, #29531, #12698, #10040, #19549, #26579, #10347, #12385, #5358, #989, #7708, #10500, #29378 ),
 .UNSPECIFIED., .F., .F.,
 ( 4, 2, 2, 2, 2, 2, 2, 2, 2, 2, 2, 2, 2, 2, 2, 4 ),
 ( 0.1181738554856288231, 0.1242296842490394210, 0.1257436414398920843, 0.1272575986307447338, 0.1302855130124500327, 0.1363413417758606305, 0.1378552989667132800, 0.1393692561575659017, 0.1423971705392711729, 0.1484529993026817429, 0.1514809136843869863, 0.1545088280660922853, 0.1605646568295027998, 0.1620786140203554493, 0.1635925712112080710, 0.1666204855929133422 ),
 .UNSPECIFIED. ) ;
#30563=CARTESIAN_POINT ( 'NONE',  ( 9.980880902826429590, -37.95465284280806628, 34.49999999999999289 ) ) ;
#30569=FACE_BOUND ( 'NONE', #12255, .T. ) ;
#30572=CARTESIAN_POINT ( 'NONE',  ( -9.746783745056944781, 38.02984302254633064, 27.50000000000000711 ) ) ;
#30588=CARTESIAN_POINT ( 'NONE',  ( 32.64610052339413926, -16.83154060456821810, 27.50000000000001421 ) ) ;
#30595=ORIENTED_EDGE ( 'NONE', *, *, #6521, .T. ) ;
#30607=CARTESIAN_POINT ( 'NONE',  ( 15.21181506329994804, -34.29657048623970894, 37.49999999996318678 ) ) ;
#30609=EDGE_LOOP ( 'NONE', ( #11290, #12301, #30023, #23012 ) ) ;
#30626=CARTESIAN_POINT ( 'NONE',  ( -24.35970437652574105, 13.37404834226503247, -16.55003854064094426 ) ) ;
#30628=VERTEX_POINT ( 'NONE', #2972 ) ;
#30630=B_SPLINE_CURVE_WITH_KNOTS ( 'NONE', 3,
 ( #3109, #19481, #24465, #22276 ),
 .UNSPECIFIED., .F., .F.,
 ( 4, 4 ),
 ( 3.018024802580205417E-07, 0.007932103453629119755 ),
 .UNSPECIFIED. ) ;
#30651=CARTESIAN_POINT ( 'NONE',  ( -38.44186125115789565, 7.193762128604462625, 32.05965621367656837 ) ) ;
#30680=ORIENTED_EDGE ( 'NONE', *, *, #6527, .F. ) ;
#30698=DIRECTION ( 'NONE',  ( 1.000000000000000000, 0.000000000000000000, -0.000000000000000000 ) ) ;
#30715=CARTESIAN_POINT ( 'NONE',  ( 0.000000000000000000, 0.000000000000000000, 27.50000000000000355 ) ) ;
#30719=EDGE_CURVE ( 'NONE', #438, #22753, #28099, .T. ) ;
#30722=CARTESIAN_POINT ( 'NONE',  ( 35.45878215871448447, 7.046087300365224237, 34.64822579837520777 ) ) ;
#30736=CARTESIAN_POINT ( 'NONE',  ( -0.8633855750855333744, -42.50000000000000000, 28.83974596215560737 ) ) ;
#30739=AXIS2_PLACEMENT_3D ( 'NONE', #23724, #19206, #12195 ) ;
#30741=CARTESIAN_POINT ( 'NONE',  ( 35.89013898050658469, 3.144164291784017795, 27.50000000000000000 ) ) ;
#30750=CARTESIAN_POINT ( 'NONE',  ( -31.79271162922631078, 14.90794587988477637, 39.88583012296479779 ) ) ;
#30770=CARTESIAN_POINT ( 'NONE',  ( 37.50556493705014560, -0.1197015986419610323, 37.50000000002331291 ) ) ;
#30787=ORIENTED_EDGE ( 'NONE', *, *, #21635, .F. ) ;
#30798=CARTESIAN_POINT ( 'NONE',  ( -23.08991993893192785, -11.27014480227852644, 49.30668222215589225 ) ) ;
#30806=LINE ( 'NONE', #11337, #16887 ) ;
#30816=VECTOR ( 'NONE', #23011, 1000.000000000000000 ) ;
#30818=CARTESIAN_POINT ( 'NONE',  ( -35.03120574897558726, 13.44240695278457309, 37.49999999996620659 ) ) ;
#30819=EDGE_LOOP ( 'NONE', ( #4904, #18939, #10846, #26634, #20029, #13074 ) ) ;
#30836=VECTOR ( 'NONE', #22946, 1000.000000000000000 ) ;
#30880=COLOUR_RGB('Light Blue',0.38,0.62,0.78);
#30881=FILL_AREA_STYLE_COLOUR('',#30880);
#30882=FILL_AREA_STYLE('',(#30881));
#30883=SURFACE_STYLE_FILL_AREA(#30882);
#30884=SURFACE_SIDE_STYLE('',(#30883));
#30885=SURFACE_STYLE_USAGE(.BOTH.,#30884);
#30886=PRESENTATION_STYLE_ASSIGNMENT((#30885));
ENDSEC;
END-ISO-10303-21;
